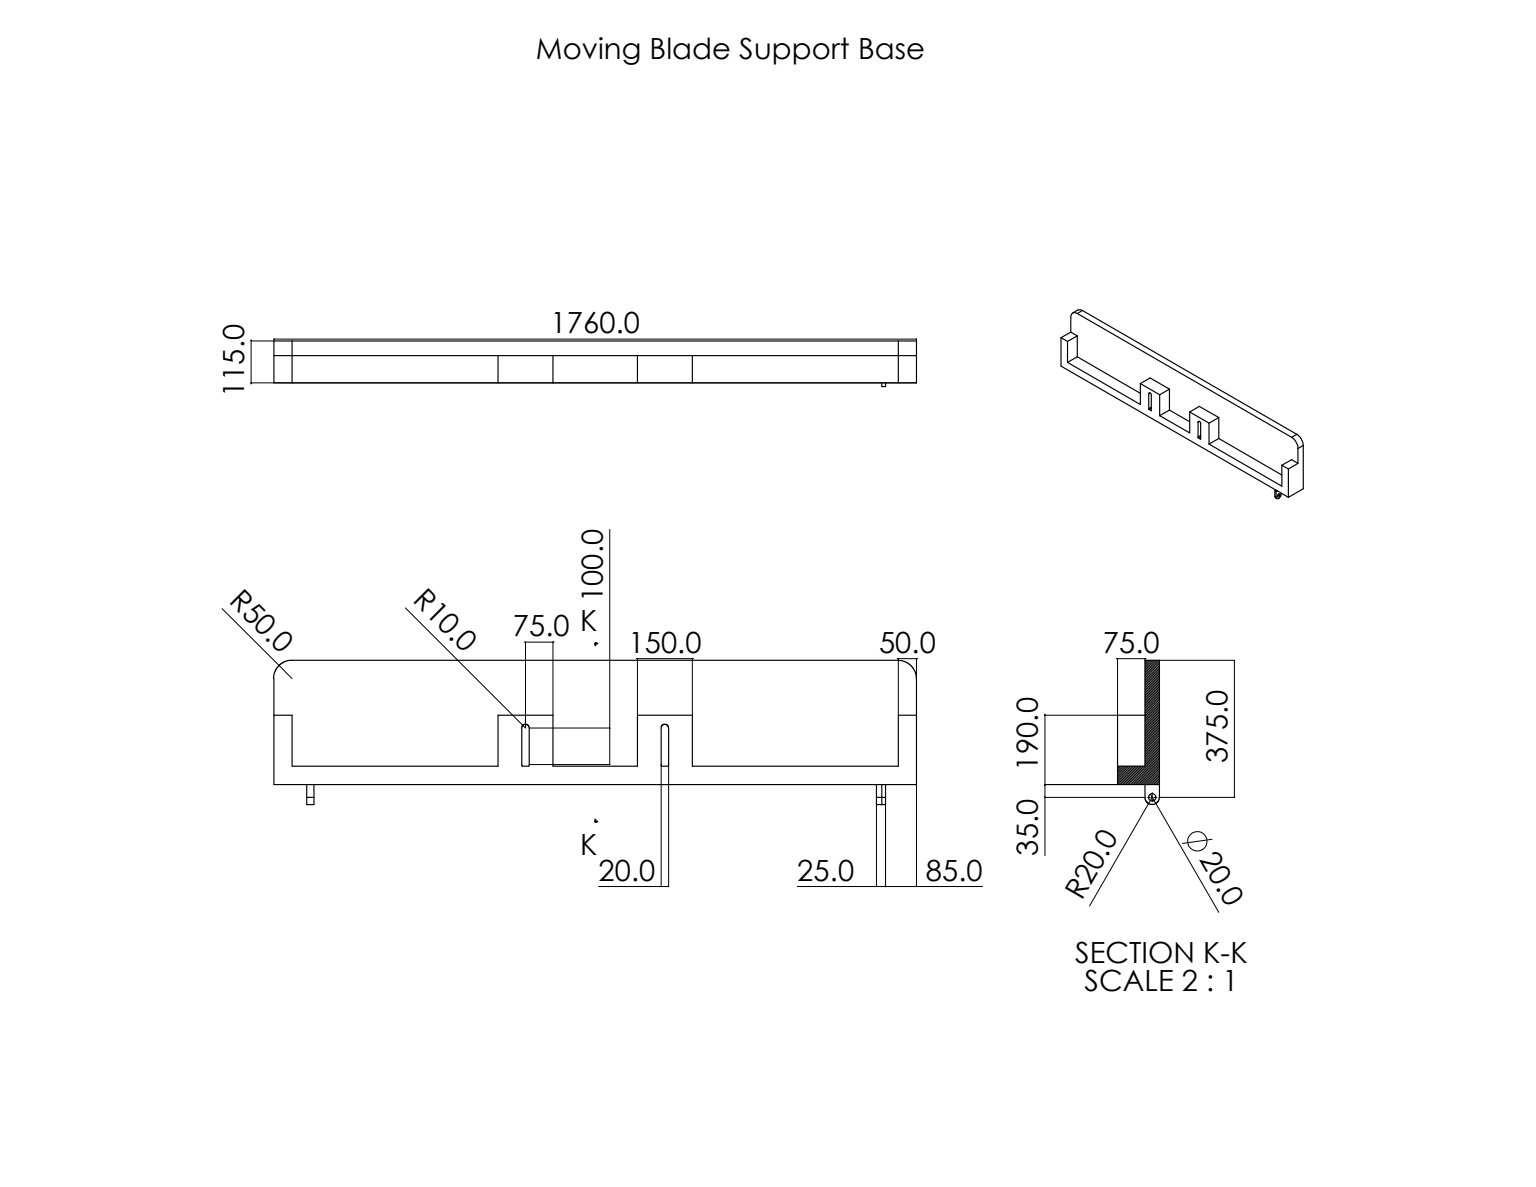
ISO-10303-21;
HEADER;
FILE_DESCRIPTION (('STEP AP214'),
    '1' );
FILE_NAME ('Moving Blade Support Base.step',
    '2026-10-21T17:07:05',
    ( '' ),
    ( '' ),
    'SwSTEP 2.0',
    'SolidWorks 2025',
    '' );
FILE_SCHEMA (( 'AUTOMOTIVE_DESIGN' ));
ENDSEC;

DATA;
#66=VERTEX_POINT ( 'NONE', #43052 ) ;
#76=DIRECTION ( 'NONE',  ( 1.000000000000000000, -5.551115123125783688E-16, 0.000000000000000000 ) ) ;
#92=DIRECTION ( 'NONE',  ( -1.000000000000000000, 0.000000000000000000, 0.000000000000000000 ) ) ;
#114=EDGE_CURVE ( 'NONE', #22938, #120, #8459, .T. ) ;
#120=VERTEX_POINT ( 'NONE', #34001 ) ;
#189=ADVANCED_FACE ( 'NONE', ( #37479 ), #13000, .F. ) ;
#193=CARTESIAN_POINT ( 'NONE',  ( -879.9999999999992042, 529.9999999999997726, -360.0000000000000000 ) ) ;
#205=EDGE_LOOP ( 'NONE', ( #30686, #19358, #44949, #34895 ) ) ;
#289=EDGE_LOOP ( 'NONE', ( #32622, #40266, #14008, #33528 ) ) ;
#307=DIRECTION ( 'NONE',  ( 1.000000000000000000, 0.000000000000000000, -0.000000000000000000 ) ) ;
#369=CARTESIAN_POINT ( 'NONE',  ( 200.7583438952259485, 394.6698570112193920, -274.9999999999999432 ) ) ;
#380=VECTOR ( 'NONE', #7221, 1000.000000000000000 ) ;
#396=AXIS2_PLACEMENT_3D ( 'NONE', #5672, #19302, #1519 ) ;
#398=CARTESIAN_POINT ( 'NONE',  ( -769.9999999999992042, 205.0000000000000568, -329.9999999999999432 ) ) ;
#404=FACE_OUTER_BOUND ( 'NONE', #21934, .T. ) ;
#412=VECTOR ( 'NONE', #33820, 1000.000000000000000 ) ;
#435=AXIS2_PLACEMENT_3D ( 'NONE', #25066, #43082, #39180 ) ;
#520=VECTOR ( 'NONE', #16329, 1000.000000000000000 ) ;
#539=ORIENTED_EDGE ( 'NONE', *, *, #26142, .F. ) ;
#553=LINE ( 'NONE', #7485, #44537 ) ;
#616=LINE ( 'NONE', #11017, #6169 ) ;
#637=VERTEX_POINT ( 'NONE', #20374 ) ;
#689=EDGE_CURVE ( 'NONE', #12562, #45491, #45323, .T. ) ;
#735=LINE ( 'NONE', #4212, #45701 ) ;
#784=CARTESIAN_POINT ( 'NONE',  ( 1238.921997096861332, 430.0000000000002842, -320.0000000000000568 ) ) ;
#829=LINE ( 'NONE', #22074, #26924 ) ;
#847=LINE ( 'NONE', #398, #9226 ) ;
#856=ORIENTED_EDGE ( 'NONE', *, *, #1291, .T. ) ;
#876=DIRECTION ( 'NONE',  ( -0.000000000000000000, -0.000000000000000000, 1.000000000000000000 ) ) ;
#879=DIRECTION ( 'NONE',  ( -0.000000000000000000, 1.000000000000000000, -0.000000000000000000 ) ) ;
#904=ORIENTED_EDGE ( 'NONE', *, *, #41975, .F. ) ;
#921=ORIENTED_EDGE ( 'NONE', *, *, #22135, .T. ) ;
#945=DIRECTION ( 'NONE',  ( 1.000000000000000000, 0.000000000000000000, 0.000000000000000000 ) ) ;
#983=FACE_OUTER_BOUND ( 'NONE', #35453, .T. ) ;
#1014=EDGE_CURVE ( 'NONE', #33458, #19810, #12588, .T. ) ;
#1053=CARTESIAN_POINT ( 'NONE',  ( -829.9999999999992042, 529.9999999999997726, -244.9999999999999716 ) ) ;
#1065=DIRECTION ( 'NONE',  ( 0.000000000000000000, 0.000000000000000000, 1.000000000000000000 ) ) ;
#1108=FACE_OUTER_BOUND ( 'NONE', #17628, .T. ) ;
#1137=AXIS2_PLACEMENT_3D ( 'NONE', #35687, #24841, #32239 ) ;
#1145=ORIENTED_EDGE ( 'NONE', *, *, #10271, .T. ) ;
#1157=ORIENTED_EDGE ( 'NONE', *, *, #3258, .T. ) ;
#1172=DIRECTION ( 'NONE',  ( 0.000000000000000000, 0.000000000000000000, -1.000000000000000000 ) ) ;
#1228=DIRECTION ( 'NONE',  ( 0.000000000000000000, 0.000000000000000000, -1.000000000000000000 ) ) ;
#1241=EDGE_LOOP ( 'NONE', ( #15487, #34240, #2964, #23570 ) ) ;
#1291=EDGE_CURVE ( 'NONE', #23098, #22606, #40548, .T. ) ;
#1294=DIRECTION ( 'NONE',  ( -0.000000000000000000, -4.857225732735055920E-15, 1.000000000000000000 ) ) ;
#1337=CARTESIAN_POINT ( 'NONE',  ( -769.9999999999992042, 205.0000000000000568, -339.9999999999999432 ) ) ;
#1348=VECTOR ( 'NONE', #24622, 1000.000000000000000 ) ;
#1386=FACE_OUTER_BOUND ( 'NONE', #24531, .T. ) ;
#1403=CARTESIAN_POINT ( 'NONE',  ( 1238.921997096861332, 240.0000000000000568, -244.9999999999999716 ) ) ;
#1470=CARTESIAN_POINT ( 'NONE',  ( -769.9999999999992042, 240.0000000000000568, -319.9999999999999432 ) ) ;
#1519=DIRECTION ( 'NONE',  ( 0.000000000000000000, 1.000000000000000000, 3.700743415417198493E-16 ) ) ;
#1552=CARTESIAN_POINT ( 'NONE',  ( 355.8971257818259915, 290.0000000000001137, -320.0000000000000568 ) ) ;
#1553=PLANE ( 'NONE',  #16394 ) ;
#1558=ADVANCED_FACE ( 'NONE', ( #21564 ), #18355, .F. ) ;
#1596=ORIENTED_EDGE ( 'NONE', *, *, #2120, .T. ) ;
#1603=PLANE ( 'NONE',  #28511 ) ;
#1607=ORIENTED_EDGE ( 'NONE', *, *, #1291, .F. ) ;
#1636=CARTESIAN_POINT ( 'NONE',  ( 1238.921997096861332, 430.0000000000002842, -244.9999999999999716 ) ) ;
#1637=VERTEX_POINT ( 'NONE', #36337 ) ;
#1647=VECTOR ( 'NONE', #23247, 1000.000000000000000 ) ;
#1656=VERTEX_POINT ( 'NONE', #25720 ) ;
#1673=AXIS2_PLACEMENT_3D ( 'NONE', #6623, #14021, #14713 ) ;
#1683=ADVANCED_FACE ( 'NONE', ( #32198 ), #25251, .F. ) ;
#1700=ORIENTED_EDGE ( 'NONE', *, *, #30911, .T. ) ;
#1702=DIRECTION ( 'NONE',  ( 1.000000000000000000, 0.000000000000000000, 0.000000000000000000 ) ) ;
#1725=CARTESIAN_POINT ( 'NONE',  ( 789.9999999999992042, 205.0000000000000568, -339.9999999999999432 ) ) ;
#1735=EDGE_CURVE ( 'NONE', #2122, #26522, #22240, .T. ) ;
#1748=ORIENTED_EDGE ( 'NONE', *, *, #16779, .F. ) ;
#1785=DIRECTION ( 'NONE',  ( 1.000000000000000000, 0.000000000000000000, -0.000000000000000000 ) ) ;
#1804=EDGE_LOOP ( 'NONE', ( #9462, #35099, #17743, #26253, #8483, #37145 ) ) ;
#1822=AXIS2_PLACEMENT_3D ( 'NONE', #15835, #9132, #36861 ) ;
#1864=ORIENTED_EDGE ( 'NONE', *, *, #14216, .T. ) ;
#1876=ORIENTED_EDGE ( 'NONE', *, *, #25151, .T. ) ;
#1966=VECTOR ( 'NONE', #876, 1000.000000000000000 ) ;
#1986=AXIS2_PLACEMENT_3D ( 'NONE', #13107, #16800, #33423 ) ;
#1992=ORIENTED_EDGE ( 'NONE', *, *, #34285, .F. ) ;
#2027=DIRECTION ( 'NONE',  ( 0.000000000000000000, 0.000000000000000000, 1.000000000000000000 ) ) ;
#2035=ORIENTED_EDGE ( 'NONE', *, *, #26712, .F. ) ;
#2077=DIRECTION ( 'NONE',  ( 0.000000000000000000, 0.000000000000000000, -1.000000000000000000 ) ) ;
#2120=EDGE_CURVE ( 'NONE', #38502, #44613, #35364, .T. ) ;
#2122=VERTEX_POINT ( 'NONE', #30995 ) ;
#2134=ADVANCED_FACE ( 'NONE', ( #45556 ), #45093, .F. ) ;
#2152=CARTESIAN_POINT ( 'NONE',  ( 180.7583438952258348, 394.6698570112193920, -274.9999999999999432 ) ) ;
#2169=PLANE ( 'NONE',  #26255 ) ;
#2178=CARTESIAN_POINT ( 'NONE',  ( 265.7583438952258916, 430.0000000000002842, -244.9999999999999716 ) ) ;
#2191=LINE ( 'NONE', #16283, #28287 ) ;
#2255=VERTEX_POINT ( 'NONE', #13451 ) ;
#2316=( GEOMETRIC_REPRESENTATION_CONTEXT ( 3 ) GLOBAL_UNCERTAINTY_ASSIGNED_CONTEXT ( ( #45060 ) ) GLOBAL_UNIT_ASSIGNED_CONTEXT ( ( #37692, #10198, #13223 ) ) REPRESENTATION_CONTEXT ( 'NONE', 'WORKASPACE' ) );
#2317=DIRECTION ( 'NONE',  ( 0.000000000000000000, -0.000000000000000000, 1.000000000000000000 ) ) ;
#2321=ORIENTED_EDGE ( 'NONE', *, *, #12855, .F. ) ;
#2355=DIRECTION ( 'NONE',  ( 0.000000000000000000, 0.000000000000000000, 1.000000000000000000 ) ) ;
#2374=ORIENTED_EDGE ( 'NONE', *, *, #14579, .T. ) ;
#2390=CARTESIAN_POINT ( 'NONE',  ( -200.7583438952258916, 294.6698570112193920, -274.9999999999999432 ) ) ;
#2394=CARTESIAN_POINT ( 'NONE',  ( -769.9999999999992042, 205.0000000000000568, -350.0000000000000000 ) ) ;
#2396=EDGE_LOOP ( 'NONE', ( #22146, #5273, #24875, #15758, #2484, #37091 ) ) ;
#2399=DIRECTION ( 'NONE',  ( -1.000000000000000000, 0.000000000000000000, 0.000000000000000000 ) ) ;
#2403=FACE_OUTER_BOUND ( 'NONE', #14861, .T. ) ;
#2473=LINE ( 'NONE', #38499, #1348 ) ;
#2484=ORIENTED_EDGE ( 'NONE', *, *, #4345, .T. ) ;
#2490=AXIS2_PLACEMENT_3D ( 'NONE', #11634, #39134, #42812 ) ;
#2569=CARTESIAN_POINT ( 'NONE',  ( 794.9999999999993179, 240.0000000000000853, -275.0000000000000000 ) ) ;
#2580=CARTESIAN_POINT ( 'NONE',  ( 784.9999999999992042, 205.0000000000000568, -255.0000000000000000 ) ) ;
#2594=VECTOR ( 'NONE', #24062, 1000.000000000000000 ) ;
#2601=FACE_OUTER_BOUND ( 'NONE', #38457, .T. ) ;
#2619=VERTEX_POINT ( 'NONE', #14363 ) ;
#2644=LINE ( 'NONE', #5407, #3910 ) ;
#2662=ADVANCED_FACE ( 'NONE', ( #28443 ), #42759, .T. ) ;
#2666=ADVANCED_FACE ( 'NONE', ( #14610 ), #43216, .F. ) ;
#2669=ORIENTED_EDGE ( 'NONE', *, *, #27519, .F. ) ;
#2752=EDGE_LOOP ( 'NONE', ( #5471, #20327, #25171, #15457 ) ) ;
#2797=ORIENTED_EDGE ( 'NONE', *, *, #18532, .T. ) ;
#2850=( NAMED_UNIT ( * ) PLANE_ANGLE_UNIT ( ) SI_UNIT ( $, .RADIAN. ) );
#2853=ORIENTED_EDGE ( 'NONE', *, *, #4945, .F. ) ;
#2878=FACE_OUTER_BOUND ( 'NONE', #35462, .T. ) ;
#2898=ADVANCED_FACE ( 'NONE', ( #5539, #37640, #18973 ), #40216, .F. ) ;
#2909=EDGE_CURVE ( 'NONE', #33022, #33694, #40657, .T. ) ;
#2964=ORIENTED_EDGE ( 'NONE', *, *, #13105, .F. ) ;
#3014=ORIENTED_EDGE ( 'NONE', *, *, #18532, .F. ) ;
#3081=DIRECTION ( 'NONE',  ( 0.000000000000000000, 0.000000000000000000, -1.000000000000000000 ) ) ;
#3082=DIRECTION ( 'NONE',  ( -0.000000000000000000, -0.000000000000000000, 1.000000000000000000 ) ) ;
#3087=VERTEX_POINT ( 'NONE', #20084 ) ;
#3094=LINE ( 'NONE', #34515, #5316 ) ;
#3171=VERTEX_POINT ( 'NONE', #6468 ) ;
#3254=CIRCLE ( 'NONE', #2490, 10.00000000000000888 ) ;
#3258=EDGE_CURVE ( 'NONE', #37112, #36817, #13621, .T. ) ;
#3270=AXIS2_PLACEMENT_3D ( 'NONE', #10948, #20633, #307 ) ;
#3325=EDGE_LOOP ( 'NONE', ( #12467, #24130 ) ) ;
#3330=DIRECTION ( 'NONE',  ( -1.000000000000000000, 0.000000000000000000, 0.000000000000000000 ) ) ;
#3343=CARTESIAN_POINT ( 'NONE',  ( 180.7583438952260622, 239.9999999999991473, -244.9999999999999716 ) ) ;
#3384=ORIENTED_EDGE ( 'NONE', *, *, #14831, .F. ) ;
#3479=EDGE_CURVE ( 'NONE', #34504, #21916, #14994, .T. ) ;
#3487=AXIS2_PLACEMENT_3D ( 'NONE', #27406, #9632, #8946 ) ;
#3553=ORIENTED_EDGE ( 'NONE', *, *, #6505, .F. ) ;
#3570=DIRECTION ( 'NONE',  ( 0.000000000000000000, 0.000000000000000000, -1.000000000000000000 ) ) ;
#3595=ORIENTED_EDGE ( 'NONE', *, *, #14216, .F. ) ;
#3605=AXIS2_PLACEMENT_3D ( 'NONE', #14612, #17604, #28446 ) ;
#3661=VECTOR ( 'NONE', #15436, 1000.000000000000000 ) ;
#3682=EDGE_LOOP ( 'NONE', ( #18165, #4144, #29968, #9995, #14865, #36556 ) ) ;
#3691=CARTESIAN_POINT ( 'NONE',  ( 355.8971257818259915, 290.0000000000001137, -244.9999999999999716 ) ) ;
#3754=ORIENTED_EDGE ( 'NONE', *, *, #38002, .F. ) ;
#3763=ORIENTED_EDGE ( 'NONE', *, *, #42223, .T. ) ;
#3805=DIRECTION ( 'NONE',  ( -0.000000000000000000, -0.000000000000000000, 1.000000000000000000 ) ) ;
#3892=ORIENTED_EDGE ( 'NONE', *, *, #42510, .F. ) ;
#3894=CARTESIAN_POINT ( 'NONE',  ( -829.9999999999994316, 579.9999999999998863, -360.0000000000000000 ) ) ;
#3910=VECTOR ( 'NONE', #13045, 1000.000000000000000 ) ;
#3938=VECTOR ( 'NONE', #20737, 1000.000000000000000 ) ;
#4027=EDGE_CURVE ( 'NONE', #37165, #1637, #32526, .T. ) ;
#4085=CARTESIAN_POINT ( 'NONE',  ( -789.9999999999992042, 205.0000000000000568, -350.0000000000000000 ) ) ;
#4086=FACE_OUTER_BOUND ( 'NONE', #29358, .T. ) ;
#4112=EDGE_CURVE ( 'NONE', #32155, #33694, #39924, .T. ) ;
#4114=EDGE_CURVE ( 'NONE', #1656, #27668, #11278, .T. ) ;
#4144=ORIENTED_EDGE ( 'NONE', *, *, #30071, .T. ) ;
#4202=CARTESIAN_POINT ( 'NONE',  ( -200.7583438952259485, 394.6698570112193920, -274.9999999999999432 ) ) ;
#4212=CARTESIAN_POINT ( 'NONE',  ( 794.9999999999993179, 205.0000000000000568, -274.9999999999999432 ) ) ;
#4234=ORIENTED_EDGE ( 'NONE', *, *, #22360, .F. ) ;
#4253=DIRECTION ( 'NONE',  ( 0.000000000000000000, 0.000000000000000000, 1.000000000000000000 ) ) ;
#4345=EDGE_CURVE ( 'NONE', #66, #19810, #34259, .T. ) ;
#4385=EDGE_CURVE ( 'NONE', #42899, #637, #19732, .T. ) ;
#4463=VERTEX_POINT ( 'NONE', #37740 ) ;
#4471=ORIENTED_EDGE ( 'NONE', *, *, #27831, .T. ) ;
#4532=LINE ( 'NONE', #22295, #34179 ) ;
#4546=ORIENTED_EDGE ( 'NONE', *, *, #26712, .T. ) ;
#4581=EDGE_CURVE ( 'NONE', #22016, #14103, #43589, .T. ) ;
#4627=EDGE_LOOP ( 'NONE', ( #36019, #24779, #36652, #33925, #45163, #24094 ) ) ;
#4685=DIRECTION ( 'NONE',  ( 1.000000000000000000, 0.000000000000000000, 0.000000000000000000 ) ) ;
#4731=ORIENTED_EDGE ( 'NONE', *, *, #1735, .F. ) ;
#4737=LINE ( 'NONE', #25067, #39541 ) ;
#4746=LINE ( 'NONE', #39656, #17406 ) ;
#4767=CARTESIAN_POINT ( 'NONE',  ( 1238.921997096861332, 240.0000000000000568, -244.9999999999999716 ) ) ;
#4776=EDGE_LOOP ( 'NONE', ( #38412, #25645 ) ) ;
#4803=LINE ( 'NONE', #26272, #24105 ) ;
#4804=DIRECTION ( 'NONE',  ( 1.000000000000000000, 0.000000000000000000, -0.000000000000000000 ) ) ;
#4815=AXIS2_PLACEMENT_3D ( 'NONE', #27835, #17202, #41930 ) ;
#4849=ORIENTED_EDGE ( 'NONE', *, *, #38917, .F. ) ;
#4857=ORIENTED_EDGE ( 'NONE', *, *, #3479, .F. ) ;
#4871=DIRECTION ( 'NONE',  ( -0.000000000000000000, -0.000000000000000000, 1.000000000000000000 ) ) ;
#4877=ADVANCED_FACE ( 'NONE', ( #21106 ), #42118, .T. ) ;
#4945=EDGE_CURVE ( 'NONE', #40516, #41324, #35818, .T. ) ;
#4955=ORIENTED_EDGE ( 'NONE', *, *, #28981, .F. ) ;
#4986=CARTESIAN_POINT ( 'NONE',  ( -265.7583438952258916, 430.0000000000002842, -244.9999999999999716 ) ) ;
#5011=EDGE_LOOP ( 'NONE', ( #3763, #40780, #25792, #15417 ) ) ;
#5037=CARTESIAN_POINT ( 'NONE',  ( -200.7583438952259485, 394.6698570112193920, -274.9999999999999432 ) ) ;
#5113=EDGE_CURVE ( 'NONE', #11672, #33458, #33310, .T. ) ;
#5137=ORIENTED_EDGE ( 'NONE', *, *, #25151, .F. ) ;
#5143=DIRECTION ( 'NONE',  ( -1.000000000000000000, -0.000000000000000000, -0.000000000000000000 ) ) ;
#5214=FACE_OUTER_BOUND ( 'NONE', #22702, .T. ) ;
#5223=ORIENTED_EDGE ( 'NONE', *, *, #1014, .T. ) ;
#5273=ORIENTED_EDGE ( 'NONE', *, *, #37945, .T. ) ;
#5274=ORIENTED_EDGE ( 'NONE', *, *, #22162, .T. ) ;
#5312=LINE ( 'NONE', #5543, #10273 ) ;
#5316=VECTOR ( 'NONE', #28249, 1000.000000000000000 ) ;
#5357=CARTESIAN_POINT ( 'NONE',  ( 794.9999999999993179, 239.9999999999998863, -235.0000000000000000 ) ) ;
#5380=CYLINDRICAL_SURFACE ( 'NONE', #27823, 20.00000000000001776 ) ;
#5381=ORIENTED_EDGE ( 'NONE', *, *, #14831, .T. ) ;
#5389=VERTEX_POINT ( 'NONE', #44381 ) ;
#5395=VERTEX_POINT ( 'NONE', #37913 ) ;
#5407=CARTESIAN_POINT ( 'NONE',  ( 769.9999999999992042, 240.0000000000000568, -319.9999999999999432 ) ) ;
#5428=PLANE ( 'NONE',  #396 ) ;
#5463=CARTESIAN_POINT ( 'NONE',  ( -829.9999999999992042, 290.0000000000001137, -244.9999999999999716 ) ) ;
#5471=ORIENTED_EDGE ( 'NONE', *, *, #42213, .F. ) ;
#5534=AXIS2_PLACEMENT_3D ( 'NONE', #41405, #23598, #27312 ) ;
#5539=FACE_BOUND ( 'NONE', #4627, .T. ) ;
#5543=CARTESIAN_POINT ( 'NONE',  ( 265.7583438952258916, 430.0000000000002842, -320.0000000000000000 ) ) ;
#5563=FACE_OUTER_BOUND ( 'NONE', #6612, .T. ) ;
#5593=CIRCLE ( 'NONE', #34347, 50.00000000000004263 ) ;
#5618=LINE ( 'NONE', #2152, #15309 ) ;
#5623=VECTOR ( 'NONE', #27450, 1000.000000000000000 ) ;
#5634=DIRECTION ( 'NONE',  ( -0.000000000000000000, 1.586032892321651891E-15, 1.000000000000000000 ) ) ;
#5644=CYLINDRICAL_SURFACE ( 'NONE', #32254, 50.00000000000004263 ) ;
#5660=VECTOR ( 'NONE', #41163, 1000.000000000000000 ) ;
#5672=CARTESIAN_POINT ( 'NONE',  ( 1238.921997096861332, 579.9999999999998863, -320.0000000000000000 ) ) ;
#5711=LINE ( 'NONE', #16106, #19361 ) ;
#5723=ORIENTED_EDGE ( 'NONE', *, *, #38818, .F. ) ;
#5754=EDGE_LOOP ( 'NONE', ( #16476, #10279, #856, #4471 ) ) ;
#5826=AXIS2_PLACEMENT_3D ( 'NONE', #9700, #16399, #44345 ) ;
#5873=DIRECTION ( 'NONE',  ( -1.000000000000000000, -0.000000000000000000, -0.000000000000000000 ) ) ;
#5902=ORIENTED_EDGE ( 'NONE', *, *, #24394, .F. ) ;
#5908=ORIENTED_EDGE ( 'NONE', *, *, #40798, .F. ) ;
#5926=PLANE ( 'NONE',  #21172 ) ;
#5947=DIRECTION ( 'NONE',  ( 0.000000000000000000, -0.000000000000000000, -1.000000000000000000 ) ) ;
#5991=DIRECTION ( 'NONE',  ( -0.000000000000000000, 1.000000000000000000, -1.586032892321652088E-15 ) ) ;
#6069=VECTOR ( 'NONE', #20486, 1000.000000000000000 ) ;
#6071=DIRECTION ( 'NONE',  ( 0.000000000000000000, 0.000000000000000000, -1.000000000000000000 ) ) ;
#6075=DIRECTION ( 'NONE',  ( 1.000000000000000000, 0.000000000000000000, 0.000000000000000000 ) ) ;
#6080=VECTOR ( 'NONE', #21557, 1000.000000000000000 ) ;
#6100=DIRECTION ( 'NONE',  ( 0.000000000000000000, -0.000000000000000000, -1.000000000000000000 ) ) ;
#6109=LINE ( 'NONE', #3343, #30527 ) ;
#6152=VECTOR ( 'NONE', #6590, 1000.000000000000000 ) ;
#6166=CARTESIAN_POINT ( 'NONE',  ( -879.9999999999992042, 529.9999999999997726, -320.0000000000000000 ) ) ;
#6169=VECTOR ( 'NONE', #25084, 1000.000000000000000 ) ;
#6188=LINE ( 'NONE', #17048, #15072 ) ;
#6217=CIRCLE ( 'NONE', #40164, 20.00000000000001776 ) ;
#6246=CARTESIAN_POINT ( 'NONE',  ( 355.8971257818259915, 290.0000000000001137, -244.9999999999999716 ) ) ;
#6263=CARTESIAN_POINT ( 'NONE',  ( 829.9999999999992042, -600.0000000000000000, -320.0000000000000568 ) ) ;
#6282=VECTOR ( 'NONE', #33387, 1000.000000000000000 ) ;
#6286=EDGE_CURVE ( 'NONE', #36310, #21150, #26154, .T. ) ;
#6312=( NAMED_UNIT ( * ) SI_UNIT ( $, .STERADIAN. ) SOLID_ANGLE_UNIT ( ) );
#6333=FACE_BOUND ( 'NONE', #3325, .T. ) ;
#6374=ADVANCED_FACE ( 'NONE', ( #2878, #6567 ), #21116, .F. ) ;
#6383=VERTEX_POINT ( 'NONE', #41914 ) ;
#6452=DIRECTION ( 'NONE',  ( 0.000000000000000000, 0.000000000000000000, -1.000000000000000000 ) ) ;
#6467=LINE ( 'NONE', #17307, #41700 ) ;
#6468=CARTESIAN_POINT ( 'NONE',  ( -879.9999999999992042, 430.0000000000002842, -320.0000000000000568 ) ) ;
#6491=AXIS2_PLACEMENT_3D ( 'NONE', #40901, #32850, #9271 ) ;
#6505=EDGE_CURVE ( 'NONE', #8476, #15857, #24555, .T. ) ;
#6527=DIRECTION ( 'NONE',  ( 0.000000000000000000, 0.000000000000000000, 1.000000000000000000 ) ) ;
#6536=VERTEX_POINT ( 'NONE', #41685 ) ;
#6546=VECTOR ( 'NONE', #14134, 1000.000000000000000 ) ;
#6567=FACE_BOUND ( 'NONE', #38886, .T. ) ;
#6590=DIRECTION ( 'NONE',  ( -0.000000000000000000, -1.000000000000000000, -0.000000000000000000 ) ) ;
#6607=EDGE_CURVE ( 'NONE', #19810, #3171, #35887, .T. ) ;
#6612=EDGE_LOOP ( 'NONE', ( #15855, #29638, #34728, #12062 ) ) ;
#6616=VECTOR ( 'NONE', #38203, 1000.000000000000000 ) ;
#6623=CARTESIAN_POINT ( 'NONE',  ( 190.7583438952258916, 294.6698570112193920, -244.9999999999999716 ) ) ;
#6674=EDGE_LOOP ( 'NONE', ( #23150, #24484, #26874, #15076 ) ) ;
#6684=CARTESIAN_POINT ( 'NONE',  ( 784.9999999999992042, 240.0000000000000853, -275.0000000000000000 ) ) ;
#6689=CARTESIAN_POINT ( 'NONE',  ( -115.7583438952258774, 430.0000000000002842, -244.9999999999999716 ) ) ;
#6744=VECTOR ( 'NONE', #39080, 1000.000000000000000 ) ;
#6804=CARTESIAN_POINT ( 'NONE',  ( -789.9999999999992042, 205.0000000000000568, -319.9999999999999432 ) ) ;
#6842=LINE ( 'NONE', #7089, #44058 ) ;
#6894=DIRECTION ( 'NONE',  ( 0.000000000000000000, 0.000000000000000000, -1.000000000000000000 ) ) ;
#6928=VERTEX_POINT ( 'NONE', #5357 ) ;
#6933=AXIS2_PLACEMENT_3D ( 'NONE', #27413, #42413, #23702 ) ;
#6999=ORIENTED_EDGE ( 'NONE', *, *, #4385, .F. ) ;
#7012=CARTESIAN_POINT ( 'NONE',  ( 180.7583438952258916, 294.6698570112193920, -274.9999999999999432 ) ) ;
#7013=ORIENTED_EDGE ( 'NONE', *, *, #38114, .F. ) ;
#7043=VECTOR ( 'NONE', #26872, 1000.000000000000000 ) ;
#7056=LINE ( 'NONE', #42153, #20163 ) ;
#7089=CARTESIAN_POINT ( 'NONE',  ( -265.7583438952258916, 290.0000000000001705, -320.0000000000000000 ) ) ;
#7096=DIRECTION ( 'NONE',  ( -1.000000000000000000, 0.000000000000000000, 0.000000000000000000 ) ) ;
#7173=EDGE_LOOP ( 'NONE', ( #5274, #37675, #45424, #10452 ) ) ;
#7221=DIRECTION ( 'NONE',  ( -0.000000000000000000, -0.000000000000000000, 1.000000000000000000 ) ) ;
#7247=EDGE_CURVE ( 'NONE', #44144, #37112, #40704, .T. ) ;
#7261=ORIENTED_EDGE ( 'NONE', *, *, #45035, .F. ) ;
#7302=ORIENTED_EDGE ( 'NONE', *, *, #38540, .T. ) ;
#7309=DIRECTION ( 'NONE',  ( 0.000000000000000000, 0.000000000000000000, -1.000000000000000000 ) ) ;
#7310=FACE_OUTER_BOUND ( 'NONE', #16254, .T. ) ;
#7328=CARTESIAN_POINT ( 'NONE',  ( -769.9999999999992042, 205.0000000000000568, -339.9999999999999432 ) ) ;
#7333=FACE_OUTER_BOUND ( 'NONE', #5754, .T. ) ;
#7367=CARTESIAN_POINT ( 'NONE',  ( 789.9999999999992042, 205.0000000000000568, -360.0000000000000000 ) ) ;
#7373=ORIENTED_EDGE ( 'NONE', *, *, #6505, .T. ) ;
#7421=ORIENTED_EDGE ( 'NONE', *, *, #24171, .F. ) ;
#7469=VERTEX_POINT ( 'NONE', #28202 ) ;
#7473=EDGE_CURVE ( 'NONE', #12764, #32851, #24501, .T. ) ;
#7476=CARTESIAN_POINT ( 'NONE',  ( 794.9999999999993179, 239.9999999999998863, -235.0000000000000000 ) ) ;
#7485=CARTESIAN_POINT ( 'NONE',  ( 829.9999999999992042, 430.0000000000002842, -320.0000000000000568 ) ) ;
#7530=DIRECTION ( 'NONE',  ( 0.000000000000000000, 0.000000000000000000, -1.000000000000000000 ) ) ;
#7531=DIRECTION ( 'NONE',  ( -0.000000000000000000, 1.000000000000000000, 6.938893903907241197E-16 ) ) ;
#7544=DIRECTION ( 'NONE',  ( -1.000000000000000000, -8.326672684688676025E-16, 0.000000000000000000 ) ) ;
#7575=VERTEX_POINT ( 'NONE', #37695 ) ;
#7611=CARTESIAN_POINT ( 'NONE',  ( 265.7583438952258916, 290.0000000000001137, -320.0000000000000568 ) ) ;
#7747=VERTEX_POINT ( 'NONE', #35584 ) ;
#7789=AXIS2_PLACEMENT_3D ( 'NONE', #7328, #7096, #34399 ) ;
#7833=DIRECTION ( 'NONE',  ( -0.000000000000000000, 1.000000000000000000, -0.000000000000000000 ) ) ;
#7838=CIRCLE ( 'NONE', #38823, 10.00000000000000888 ) ;
#7849=DIRECTION ( 'NONE',  ( -1.000000000000000000, -0.000000000000000000, -0.000000000000000000 ) ) ;
#7937=EDGE_LOOP ( 'NONE', ( #28588, #37208, #32066, #23296 ) ) ;
#7952=LINE ( 'NONE', #43032, #8407 ) ;
#7998=DIRECTION ( 'NONE',  ( 1.000000000000000000, -0.000000000000000000, -0.000000000000000000 ) ) ;
#8057=CARTESIAN_POINT ( 'NONE',  ( -265.7583438952258916, -600.0000000000000000, -320.0000000000000000 ) ) ;
#8082=LINE ( 'NONE', #11980, #37938 ) ;
#8131=EDGE_CURVE ( 'NONE', #16382, #12764, #34405, .T. ) ;
#8171=LINE ( 'NONE', #43485, #6080 ) ;
#8204=VERTEX_POINT ( 'NONE', #38113 ) ;
#8226=CARTESIAN_POINT ( 'NONE',  ( 879.9999999999992042, 240.0000000000000568, -244.9999999999999716 ) ) ;
#8274=EDGE_CURVE ( 'NONE', #31293, #5389, #6467, .T. ) ;
#8328=VECTOR ( 'NONE', #17490, 1000.000000000000000 ) ;
#8368=ORIENTED_EDGE ( 'NONE', *, *, #26992, .F. ) ;
#8378=LINE ( 'NONE', #12070, #36619 ) ;
#8407=VECTOR ( 'NONE', #11396, 1000.000000000000000 ) ;
#8421=VERTEX_POINT ( 'NONE', #9476 ) ;
#8428=ORIENTED_EDGE ( 'NONE', *, *, #34615, .F. ) ;
#8459=CIRCLE ( 'NONE', #34244, 10.00000000000006395 ) ;
#8476=VERTEX_POINT ( 'NONE', #33204 ) ;
#8483=ORIENTED_EDGE ( 'NONE', *, *, #44416, .T. ) ;
#8503=CARTESIAN_POINT ( 'NONE',  ( 265.7583438952258916, -600.0000000000000000, -244.9999999999999716 ) ) ;
#8540=ORIENTED_EDGE ( 'NONE', *, *, #1014, .F. ) ;
#8601=ORIENTED_EDGE ( 'NONE', *, *, #23000, .T. ) ;
#8619=CARTESIAN_POINT ( 'NONE',  ( -829.9999999999992042, -600.0000000000000000, -244.9999999999995168 ) ) ;
#8644=AXIS2_PLACEMENT_3D ( 'NONE', #7476, #35628, #32182 ) ;
#8657=ORIENTED_EDGE ( 'NONE', *, *, #42213, .T. ) ;
#8665=ORIENTED_EDGE ( 'NONE', *, *, #17723, .T. ) ;
#8703=CARTESIAN_POINT ( 'NONE',  ( 1238.921997096861332, 240.0000000000000853, -360.0000000000000000 ) ) ;
#8742=CYLINDRICAL_SURFACE ( 'NONE', #18710, 10.00000000000000888 ) ;
#8871=ORIENTED_EDGE ( 'NONE', *, *, #15402, .F. ) ;
#8900=FACE_OUTER_BOUND ( 'NONE', #2396, .T. ) ;
#8920=EDGE_LOOP ( 'NONE', ( #921, #1748, #23517, #35732 ) ) ;
#8922=ADVANCED_FACE ( 'NONE', ( #13784 ), #16789, .F. ) ;
#8926=EDGE_LOOP ( 'NONE', ( #5902, #20512, #35977, #20567, #33801, #30215 ) ) ;
#8941=LINE ( 'NONE', #23470, #18218 ) ;
#8946=DIRECTION ( 'NONE',  ( 0.000000000000000000, 0.000000000000000000, -1.000000000000000000 ) ) ;
#9031=VERTEX_POINT ( 'NONE', #38034 ) ;
#9039=CIRCLE ( 'NONE', #34852, 19.99999999999998934 ) ;
#9107=CARTESIAN_POINT ( 'NONE',  ( 180.7583438952258916, 294.6698570112193920, -274.9999999999999432 ) ) ;
#9132=DIRECTION ( 'NONE',  ( -0.000000000000000000, 1.000000000000000000, 0.000000000000000000 ) ) ;
#9136=EDGE_LOOP ( 'NONE', ( #44530, #32686, #26588, #20152, #28994, #40255, #11894, #45303, #1864, #16311, #5908, #22664, #25054, #38306 ) ) ;
#9154=ORIENTED_EDGE ( 'NONE', *, *, #34274, .T. ) ;
#9166=CARTESIAN_POINT ( 'NONE',  ( 784.9999999999992042, 239.9999999999998863, -235.0000000000000000 ) ) ;
#9172=AXIS2_PLACEMENT_3D ( 'NONE', #36324, #11391, #4685 ) ;
#9182=EDGE_CURVE ( 'NONE', #44613, #25018, #20235, .T. ) ;
#9226=VECTOR ( 'NONE', #14502, 1000.000000000000000 ) ;
#9253=LINE ( 'NONE', #12265, #37540 ) ;
#9271=DIRECTION ( 'NONE',  ( 0.000000000000000000, 0.000000000000000000, 1.000000000000000000 ) ) ;
#9287=LINE ( 'NONE', #6263, #43996 ) ;
#9320=ADVANCED_FACE ( 'NONE', ( #7310 ), #14225, .F. ) ;
#9326=VECTOR ( 'NONE', #39284, 1000.000000000000000 ) ;
#9337=CARTESIAN_POINT ( 'NONE',  ( 794.9999999999993179, 240.0000000000000853, -275.0000000000000000 ) ) ;
#9354=AXIS2_PLACEMENT_3D ( 'NONE', #24545, #31714, #38428 ) ;
#9422=VECTOR ( 'NONE', #15736, 1000.000000000000000 ) ;
#9431=EDGE_CURVE ( 'NONE', #4463, #22016, #4737, .T. ) ;
#9451=ORIENTED_EDGE ( 'NONE', *, *, #30318, .F. ) ;
#9462=ORIENTED_EDGE ( 'NONE', *, *, #27723, .T. ) ;
#9473=ADVANCED_FACE ( 'NONE', ( #39644 ), #38960, .F. ) ;
#9476=CARTESIAN_POINT ( 'NONE',  ( 784.9999999999992042, 205.0000000000000568, -245.0000000000000284 ) ) ;
#9498=ORIENTED_EDGE ( 'NONE', *, *, #33454, .F. ) ;
#9540=DIRECTION ( 'NONE',  ( 0.000000000000000000, 0.000000000000000000, 1.000000000000000000 ) ) ;
#9554=VECTOR ( 'NONE', #3082, 1000.000000000000000 ) ;
#9569=ORIENTED_EDGE ( 'NONE', *, *, #43347, .F. ) ;
#9581=DIRECTION ( 'NONE',  ( -0.000000000000000000, 1.000000000000000000, -0.000000000000000000 ) ) ;
#9632=DIRECTION ( 'NONE',  ( 1.000000000000000000, 0.000000000000000000, 0.000000000000000000 ) ) ;
#9638=CARTESIAN_POINT ( 'NONE',  ( -769.9999999999992042, 205.0000000000000568, -319.9999999999999432 ) ) ;
#9674=EDGE_LOOP ( 'NONE', ( #7421, #36199, #42960, #15361 ) ) ;
#9700=CARTESIAN_POINT ( 'NONE',  ( -190.7583438952258916, 294.6698570112193920, -244.9999999999999716 ) ) ;
#9724=ADVANCED_FACE ( 'NONE', ( #22945 ), #2169, .F. ) ;
#9770=CARTESIAN_POINT ( 'NONE',  ( 180.7583438952258348, 394.6698570112193920, -274.9999999999999432 ) ) ;
#9799=LINE ( 'NONE', #16053, #25297 ) ;
#9822=EDGE_LOOP ( 'NONE', ( #5137, #2321, #44202, #36220 ) ) ;
#9901=LINE ( 'NONE', #13840, #19641 ) ;
#9949=CIRCLE ( 'NONE', #15847, 19.99999999999998934 ) ;
#9953=CIRCLE ( 'NONE', #29152, 20.00000000000001776 ) ;
#9984=EDGE_CURVE ( 'NONE', #39117, #22606, #37331, .T. ) ;
#9995=ORIENTED_EDGE ( 'NONE', *, *, #35112, .F. ) ;
#10035=FACE_OUTER_BOUND ( 'NONE', #1241, .T. ) ;
#10049=AXIS2_PLACEMENT_3D ( 'NONE', #31512, #13279, #92 ) ;
#10082=DIRECTION ( 'NONE',  ( -0.000000000000000000, 0.000000000000000000, -1.000000000000000000 ) ) ;
#10094=VECTOR ( 'NONE', #43379, 1000.000000000000000 ) ;
#10175=DIRECTION ( 'NONE',  ( 1.000000000000000000, 0.000000000000000000, 0.000000000000000000 ) ) ;
#10179=VECTOR ( 'NONE', #18760, 1000.000000000000000 ) ;
#10198=( NAMED_UNIT ( * ) PLANE_ANGLE_UNIT ( ) SI_UNIT ( $, .RADIAN. ) );
#10204=VECTOR ( 'NONE', #44836, 1000.000000000000000 ) ;
#10217=CARTESIAN_POINT ( 'NONE',  ( -180.7583438952258348, 394.6698570112193920, -274.9999999999999432 ) ) ;
#10220=VERTEX_POINT ( 'NONE', #38653 ) ;
#10226=PLANE ( 'NONE',  #38925 ) ;
#10240=CARTESIAN_POINT ( 'NONE',  ( 794.9999999999993179, 205.0000000000000568, -255.0000000000000000 ) ) ;
#10271=EDGE_CURVE ( 'NONE', #2255, #36814, #32900, .T. ) ;
#10273=VECTOR ( 'NONE', #27260, 1000.000000000000000 ) ;
#10274=CARTESIAN_POINT ( 'NONE',  ( 769.9999999999992042, 205.0000000000000568, -339.9999999999999432 ) ) ;
#10276=ADVANCED_FACE ( 'NONE', ( #45361 ), #41895, .T. ) ;
#10279=ORIENTED_EDGE ( 'NONE', *, *, #15141, .F. ) ;
#10334=ORIENTED_EDGE ( 'NONE', *, *, #43836, .T. ) ;
#10445=ORIENTED_EDGE ( 'NONE', *, *, #41975, .T. ) ;
#10452=ORIENTED_EDGE ( 'NONE', *, *, #16779, .T. ) ;
#10477=DIRECTION ( 'NONE',  ( 0.000000000000000000, -1.000000000000000000, 0.000000000000000000 ) ) ;
#10535=CARTESIAN_POINT ( 'NONE',  ( 180.7583438952258348, 394.6698570112193920, -274.9999999999999432 ) ) ;
#10564=ADVANCED_FACE ( 'NONE', ( #25704 ), #22012, .F. ) ;
#10572=ORIENTED_EDGE ( 'NONE', *, *, #37945, .F. ) ;
#10629=AXIS2_PLACEMENT_3D ( 'NONE', #32436, #25492, #42820 ) ;
#10643=CARTESIAN_POINT ( 'NONE',  ( 265.7583438952258916, 290.0000000000001137, -244.9999999999999716 ) ) ;
#10657=VECTOR ( 'NONE', #43929, 1000.000000000000000 ) ;
#10662=DIRECTION ( 'NONE',  ( 0.000000000000000000, 0.000000000000000000, -1.000000000000000000 ) ) ;
#10715=CARTESIAN_POINT ( 'NONE',  ( 1238.921997096861332, 430.0000000000002842, -320.0000000000000568 ) ) ;
#10756=ORIENTED_EDGE ( 'NONE', *, *, #24413, .F. ) ;
#10829=CARTESIAN_POINT ( 'NONE',  ( 175.6195620086261613, 290.0000000000001137, -320.0000000000000568 ) ) ;
#10884=EDGE_CURVE ( 'NONE', #1637, #45115, #8378, .T. ) ;
#10898=CARTESIAN_POINT ( 'NONE',  ( 1238.921997096861332, 240.0000000000000568, -244.9999999999999716 ) ) ;
#10932=EDGE_LOOP ( 'NONE', ( #16729, #35225, #3892, #20497 ) ) ;
#10944=CARTESIAN_POINT ( 'NONE',  ( 200.7583438952259485, 394.6698570112193920, -274.9999999999999432 ) ) ;
#10948=CARTESIAN_POINT ( 'NONE',  ( 190.7583438952259485, 394.6698570112193920, -274.9999999999999432 ) ) ;
#10974=CARTESIAN_POINT ( 'NONE',  ( -115.7583438952258774, 430.0000000000002842, -244.9999999999999716 ) ) ;
#11017=CARTESIAN_POINT ( 'NONE',  ( 769.9999999999992042, 240.0000000000000568, -319.9999999999999432 ) ) ;
#11091=CARTESIAN_POINT ( 'NONE',  ( 794.9999999999993179, 205.0000000000000568, -265.0000000000000000 ) ) ;
#11092=ORIENTED_EDGE ( 'NONE', *, *, #22976, .T. ) ;
#11140=EDGE_CURVE ( 'NONE', #15121, #26522, #13214, .T. ) ;
#11150=EDGE_CURVE ( 'NONE', #14103, #7469, #9287, .T. ) ;
#11220=FACE_OUTER_BOUND ( 'NONE', #29159, .T. ) ;
#11225=LINE ( 'NONE', #369, #17442 ) ;
#11251=DIRECTION ( 'NONE',  ( -1.000000000000000000, -0.000000000000000000, -0.000000000000000000 ) ) ;
#11266=VERTEX_POINT ( 'NONE', #7367 ) ;
#11267=PRODUCT_CONTEXT ( 'NONE', #19019, 'mechanical' ) ;
#11278=LINE ( 'NONE', #42460, #11468 ) ;
#11336=ORIENTED_EDGE ( 'NONE', *, *, #44934, .F. ) ;
#11350=DIRECTION ( 'NONE',  ( 0.000000000000000000, 0.000000000000000000, 1.000000000000000000 ) ) ;
#11354=ADVANCED_FACE ( 'NONE', ( #22125 ), #36437, .F. ) ;
#11371=LINE ( 'NONE', #14388, #20500 ) ;
#11391=DIRECTION ( 'NONE',  ( 0.000000000000000000, -0.000000000000000000, -1.000000000000000000 ) ) ;
#11396=DIRECTION ( 'NONE',  ( -1.000000000000000000, -0.000000000000000000, -0.000000000000000000 ) ) ;
#11468=VECTOR ( 'NONE', #11513, 1000.000000000000000 ) ;
#11492=CARTESIAN_POINT ( 'NONE',  ( -115.7583438952258774, 430.0000000000002842, -320.0000000000000568 ) ) ;
#11513=DIRECTION ( 'NONE',  ( -1.000000000000000000, -0.000000000000000000, -0.000000000000000000 ) ) ;
#11532=ADVANCED_FACE ( 'NONE', ( #32999 ), #39927, .T. ) ;
#11590=DIRECTION ( 'NONE',  ( 0.000000000000000000, -0.000000000000000000, 1.000000000000000000 ) ) ;
#11611=EDGE_LOOP ( 'NONE', ( #1157, #43247, #14322, #40627, #27114 ) ) ;
#11618=EDGE_LOOP ( 'NONE', ( #25727, #21084, #38889, #43403 ) ) ;
#11634=CARTESIAN_POINT ( 'NONE',  ( 789.9999999999992042, 205.0000000000000568, -339.9999999999999432 ) ) ;
#11644=VECTOR ( 'NONE', #45117, 1000.000000000000000 ) ;
#11651=EDGE_CURVE ( 'NONE', #4463, #27157, #22571, .T. ) ;
#11672=VERTEX_POINT ( 'NONE', #14762 ) ;
#11726=EDGE_CURVE ( 'NONE', #43685, #21532, #44276, .T. ) ;
#11831=ORIENTED_EDGE ( 'NONE', *, *, #4114, .T. ) ;
#11894=ORIENTED_EDGE ( 'NONE', *, *, #18732, .F. ) ;
#11906=CYLINDRICAL_SURFACE ( 'NONE', #12706, 50.00000000000004263 ) ;
#11930=CIRCLE ( 'NONE', #28149, 10.00000000000000888 ) ;
#11931=EDGE_CURVE ( 'NONE', #11672, #8476, #30408, .T. ) ;
#11972=EDGE_CURVE ( 'NONE', #32155, #8476, #15873, .T. ) ;
#11980=CARTESIAN_POINT ( 'NONE',  ( -115.7583438952258774, 290.0000000000001705, -244.9999999999999716 ) ) ;
#12062=ORIENTED_EDGE ( 'NONE', *, *, #18732, .T. ) ;
#12070=CARTESIAN_POINT ( 'NONE',  ( -789.9999999999992042, 240.0000000000000568, -319.9999999999999432 ) ) ;
#12079=EDGE_CURVE ( 'NONE', #38375, #637, #35247, .T. ) ;
#12083=VECTOR ( 'NONE', #40338, 1000.000000000000000 ) ;
#12129=CARTESIAN_POINT ( 'NONE',  ( -829.9999999999992042, 430.0000000000002842, -319.9999999999996021 ) ) ;
#12132=DIRECTION ( 'NONE',  ( 0.000000000000000000, 0.000000000000000000, -1.000000000000000000 ) ) ;
#12164=EDGE_LOOP ( 'NONE', ( #43790, #21589, #34080, #36443 ) ) ;
#12168=AXIS2_PLACEMENT_3D ( 'NONE', #17679, #17447, #27370 ) ;
#12210=DIRECTION ( 'NONE',  ( 0.000000000000000000, -1.000000000000000000, 0.000000000000000000 ) ) ;
#12265=CARTESIAN_POINT ( 'NONE',  ( 879.9999999999992042, 579.9999999999998863, -320.0000000000000000 ) ) ;
#12268=VECTOR ( 'NONE', #25409, 1000.000000000000000 ) ;
#12283=FACE_BOUND ( 'NONE', #4776, .T. ) ;
#12294=ORIENTED_EDGE ( 'NONE', *, *, #44450, .T. ) ;
#12296=VECTOR ( 'NONE', #7833, 1000.000000000000000 ) ;
#12327=DIRECTION ( 'NONE',  ( -1.000000000000000000, 0.000000000000000000, 0.000000000000000000 ) ) ;
#12414=CARTESIAN_POINT ( 'NONE',  ( -879.9999999999992042, 579.9999999999998863, -360.0000000000000000 ) ) ;
#12422=CARTESIAN_POINT ( 'NONE',  ( 190.7583438952258916, 294.6698570112193920, -274.9999999999999432 ) ) ;
#12428=ORIENTED_EDGE ( 'NONE', *, *, #43078, .T. ) ;
#12447=VERTEX_POINT ( 'NONE', #25973 ) ;
#12463=CARTESIAN_POINT ( 'NONE',  ( 879.9999999999992042, 579.9999999999998863, -360.0000000000000000 ) ) ;
#12467=ORIENTED_EDGE ( 'NONE', *, *, #37644, .F. ) ;
#12474=CARTESIAN_POINT ( 'NONE',  ( 355.8971257818259915, 290.0000000000001137, -244.9999999999999716 ) ) ;
#12562=VERTEX_POINT ( 'NONE', #42862 ) ;
#12588=LINE ( 'NONE', #22966, #37250 ) ;
#12589=DIRECTION ( 'NONE',  ( 1.000000000000000000, -0.000000000000000000, 0.000000000000000000 ) ) ;
#12633=DIRECTION ( 'NONE',  ( 0.000000000000000000, -1.000000000000000000, 0.000000000000000000 ) ) ;
#12682=LINE ( 'NONE', #13605, #41557 ) ;
#12706=AXIS2_PLACEMENT_3D ( 'NONE', #1053, #25768, #21619 ) ;
#12736=PLANE ( 'NONE',  #37380 ) ;
#12764=VERTEX_POINT ( 'NONE', #28780 ) ;
#12802=CARTESIAN_POINT ( 'NONE',  ( 1238.921997096861332, 579.9999999999998863, -360.0000000000000000 ) ) ;
#12855=EDGE_CURVE ( 'NONE', #39585, #26480, #11225, .T. ) ;
#13000=PLANE ( 'NONE',  #5534 ) ;
#13009=ORIENTED_EDGE ( 'NONE', *, *, #39172, .F. ) ;
#13045=DIRECTION ( 'NONE',  ( 1.000000000000000000, 0.000000000000000000, 0.000000000000000000 ) ) ;
#13067=PLANE ( 'NONE',  #12168 ) ;
#13105=EDGE_CURVE ( 'NONE', #25018, #7575, #32934, .T. ) ;
#13107=CARTESIAN_POINT ( 'NONE',  ( -190.7583438952258916, 294.6698570112193920, -274.9999999999999432 ) ) ;
#13114=LINE ( 'NONE', #9638, #45250 ) ;
#13136=VERTEX_POINT ( 'NONE', #2394 ) ;
#13161=EDGE_LOOP ( 'NONE', ( #18940, #30114, #2853, #15354 ) ) ;
#13183=EDGE_CURVE ( 'NONE', #26065, #11266, #19963, .T. ) ;
#13199=PLANE ( 'NONE',  #35233 ) ;
#13214=LINE ( 'NONE', #39017, #43282 ) ;
#13223=( NAMED_UNIT ( * ) SI_UNIT ( $, .STERADIAN. ) SOLID_ANGLE_UNIT ( ) );
#13256=ORIENTED_EDGE ( 'NONE', *, *, #37668, .F. ) ;
#13263=DIRECTION ( 'NONE',  ( 0.000000000000000000, 0.000000000000000000, -1.000000000000000000 ) ) ;
#13279=DIRECTION ( 'NONE',  ( 0.000000000000000000, 0.000000000000000000, -1.000000000000000000 ) ) ;
#13329=LINE ( 'NONE', #44279, #520 ) ;
#13340=CARTESIAN_POINT ( 'NONE',  ( 190.7583438952258916, 294.6698570112193920, -244.9999999999999716 ) ) ;
#13342=DIRECTION ( 'NONE',  ( 0.000000000000000000, 0.000000000000000000, 1.000000000000000000 ) ) ;
#13350=CARTESIAN_POINT ( 'NONE',  ( 794.9999999999993179, 239.9999999999998863, -235.0000000000000000 ) ) ;
#13377=LINE ( 'NONE', #10829, #5623 ) ;
#13412=EDGE_CURVE ( 'NONE', #8421, #32576, #18929, .T. ) ;
#13414=ORIENTED_EDGE ( 'NONE', *, *, #35683, .F. ) ;
#13420=AXIS2_PLACEMENT_3D ( 'NONE', #2580, #24737, #1172 ) ;
#13451=CARTESIAN_POINT ( 'NONE',  ( 794.9999999999993179, 205.0000000000000568, -245.0000000000000284 ) ) ;
#13536=VECTOR ( 'NONE', #34578, 1000.000000000000000 ) ;
#13558=CARTESIAN_POINT ( 'NONE',  ( -199.6009925648704098, 290.0000000000001137, -274.9999999999999432 ) ) ;
#13586=DIRECTION ( 'NONE',  ( -1.000000000000000000, -0.000000000000000000, -0.000000000000000000 ) ) ;
#13604=PLANE ( 'NONE',  #32976 ) ;
#13605=CARTESIAN_POINT ( 'NONE',  ( 1238.921997096861332, 430.0000000000002842, -320.0000000000000568 ) ) ;
#13621=LINE ( 'NONE', #38556, #38732 ) ;
#13722=CARTESIAN_POINT ( 'NONE',  ( 789.9999999999992042, 205.0000000000000568, -329.9999999999999432 ) ) ;
#13727=DIRECTION ( 'NONE',  ( 0.000000000000000000, 0.000000000000000000, -1.000000000000000000 ) ) ;
#13729=VERTEX_POINT ( 'NONE', #23632 ) ;
#13746=AXIS2_PLACEMENT_3D ( 'NONE', #42113, #28019, #13263 ) ;
#13784=FACE_OUTER_BOUND ( 'NONE', #11618, .T. ) ;
#13793=CARTESIAN_POINT ( 'NONE',  ( -180.7583438952258916, 294.6698570112193920, -244.9999999999999716 ) ) ;
#13840=CARTESIAN_POINT ( 'NONE',  ( 200.7583438952259485, 394.6698570112193920, -274.9999999999999432 ) ) ;
#13877=CARTESIAN_POINT ( 'NONE',  ( 1238.921997096861332, 579.9999999999998863, -360.0000000000000000 ) ) ;
#13931=CARTESIAN_POINT ( 'NONE',  ( 794.9999999999993179, 205.0000000000000568, -255.0000000000000000 ) ) ;
#13963=DIRECTION ( 'NONE',  ( 1.000000000000000000, 0.000000000000000000, -0.000000000000000000 ) ) ;
#13990=ADVANCED_FACE ( 'NONE', ( #1386 ), #1603, .F. ) ;
#14008=ORIENTED_EDGE ( 'NONE', *, *, #28981, .T. ) ;
#14021=DIRECTION ( 'NONE',  ( 0.000000000000000000, 0.000000000000000000, -1.000000000000000000 ) ) ;
#14032=CARTESIAN_POINT ( 'NONE',  ( 794.9999999999993179, 205.0000000000000568, -255.0000000000000000 ) ) ;
#14103=VERTEX_POINT ( 'NONE', #17870 ) ;
#14134=DIRECTION ( 'NONE',  ( -5.551115123125783688E-16, 1.000000000000000000, 0.000000000000000000 ) ) ;
#14204=ORIENTED_EDGE ( 'NONE', *, *, #18199, .T. ) ;
#14216=EDGE_CURVE ( 'NONE', #26065, #45022, #44800, .T. ) ;
#14225=PLANE ( 'NONE',  #15167 ) ;
#14244=ADVANCED_FACE ( 'NONE', ( #16378 ), #37854, .F. ) ;
#14245=CARTESIAN_POINT ( 'NONE',  ( 200.7583438952258348, 240.0000000000006253, -244.9999999999999716 ) ) ;
#14254=EDGE_CURVE ( 'NONE', #41324, #38502, #44099, .T. ) ;
#14322=ORIENTED_EDGE ( 'NONE', *, *, #33474, .T. ) ;
#14363=CARTESIAN_POINT ( 'NONE',  ( -789.9999999999992042, 205.0000000000000568, -319.9999999999999432 ) ) ;
#14366=CARTESIAN_POINT ( 'NONE',  ( -789.9999999999992042, 205.0000000000000568, -360.0000000000000000 ) ) ;
#14388=CARTESIAN_POINT ( 'NONE',  ( 879.9999999999992042, 430.0000000000002842, -320.0000000000000568 ) ) ;
#14403=VECTOR ( 'NONE', #35136, 1000.000000000000000 ) ;
#14437=ADVANCED_BREP_SHAPE_REPRESENTATION ( '', ( #17465, #26858 ), #41617 ) ;
#14502=DIRECTION ( 'NONE',  ( -1.000000000000000000, 0.000000000000000000, 0.000000000000000000 ) ) ;
#14507=PLANE ( 'NONE',  #17974 ) ;
#14549=ADVANCED_FACE ( 'NONE', ( #21669 ), #13604, .F. ) ;
#14579=EDGE_CURVE ( 'NONE', #22309, #27668, #4803, .T. ) ;
#14610=FACE_OUTER_BOUND ( 'NONE', #6674, .T. ) ;
#14612=CARTESIAN_POINT ( 'NONE',  ( 1238.921997096861332, 430.0000000000002842, -320.0000000000000568 ) ) ;
#14656=DIRECTION ( 'NONE',  ( -0.000000000000000000, -0.000000000000000000, -1.000000000000000000 ) ) ;
#14713=DIRECTION ( 'NONE',  ( -1.000000000000000000, 0.000000000000000000, 0.000000000000000000 ) ) ;
#14716=EDGE_CURVE ( 'NONE', #45077, #33694, #40140, .T. ) ;
#14762=CARTESIAN_POINT ( 'NONE',  ( -829.9999999999992042, 290.0000000000001137, -244.9999999999999716 ) ) ;
#14809=CARTESIAN_POINT ( 'NONE',  ( 1238.921997096861332, 240.0000000000000568, -244.9999999999999716 ) ) ;
#14831=EDGE_CURVE ( 'NONE', #22309, #35390, #15221, .T. ) ;
#14861=EDGE_LOOP ( 'NONE', ( #1700, #28992, #22479, #8601 ) ) ;
#14865=ORIENTED_EDGE ( 'NONE', *, *, #9182, .F. ) ;
#14928=DIRECTION ( 'NONE',  ( -0.000000000000000000, 1.000000000000000000, -0.000000000000000000 ) ) ;
#14974=DIRECTION ( 'NONE',  ( 0.000000000000000000, 0.000000000000000000, -1.000000000000000000 ) ) ;
#14994=LINE ( 'NONE', #3691, #23238 ) ;
#15072=VECTOR ( 'NONE', #30913, 1000.000000000000000 ) ;
#15076=ORIENTED_EDGE ( 'NONE', *, *, #38818, .T. ) ;
#15112=EDGE_CURVE ( 'NONE', #15121, #22938, #13329, .T. ) ;
#15121=VERTEX_POINT ( 'NONE', #34336 ) ;
#15122=ADVANCED_FACE ( 'NONE', ( #20020 ), #23696, .F. ) ;
#15141=EDGE_CURVE ( 'NONE', #23098, #22342, #27815, .T. ) ;
#15157=CARTESIAN_POINT ( 'NONE',  ( 769.9999999999992042, 205.0000000000000568, -339.9999999999999432 ) ) ;
#15167=AXIS2_PLACEMENT_3D ( 'NONE', #18609, #7531, #25757 ) ;
#15184=AXIS2_PLACEMENT_3D ( 'NONE', #20150, #9540, #37710 ) ;
#15219=DIRECTION ( 'NONE',  ( 0.000000000000000000, 0.000000000000000000, 1.000000000000000000 ) ) ;
#15221=LINE ( 'NONE', #1552, #32237 ) ;
#15274=AXIS2_PLACEMENT_3D ( 'NONE', #1337, #25125, #15442 ) ;
#15309=VECTOR ( 'NONE', #29878, 1000.000000000000000 ) ;
#15323=FACE_OUTER_BOUND ( 'NONE', #28244, .T. ) ;
#15354=ORIENTED_EDGE ( 'NONE', *, *, #23000, .F. ) ;
#15361=ORIENTED_EDGE ( 'NONE', *, *, #24394, .T. ) ;
#15379=CARTESIAN_POINT ( 'NONE',  ( 1238.921997096861332, 430.0000000000002842, -244.9999999999999716 ) ) ;
#15385=DIRECTION ( 'NONE',  ( -0.000000000000000000, 1.000000000000000000, -0.000000000000000000 ) ) ;
#15399=CARTESIAN_POINT ( 'NONE',  ( 794.9999999999993179, 205.0000000000000568, -255.0000000000000000 ) ) ;
#15402=EDGE_CURVE ( 'NONE', #32155, #39971, #6842, .T. ) ;
#15409=ORIENTED_EDGE ( 'NONE', *, *, #41940, .T. ) ;
#15417=ORIENTED_EDGE ( 'NONE', *, *, #40798, .T. ) ;
#15425=ORIENTED_EDGE ( 'NONE', *, *, #30524, .F. ) ;
#15436=DIRECTION ( 'NONE',  ( -0.000000000000000000, -0.000000000000000000, 1.000000000000000000 ) ) ;
#15439=CIRCLE ( 'NONE', #41241, 10.00000000000006395 ) ;
#15442=DIRECTION ( 'NONE',  ( 0.000000000000000000, 0.000000000000000000, 1.000000000000000000 ) ) ;
#15457=ORIENTED_EDGE ( 'NONE', *, *, #43836, .F. ) ;
#15487=ORIENTED_EDGE ( 'NONE', *, *, #32318, .T. ) ;
#15490=DIRECTION ( 'NONE',  ( -1.000000000000000000, 0.000000000000000000, 0.000000000000000000 ) ) ;
#15491=CARTESIAN_POINT ( 'NONE',  ( -769.9999999999992042, 240.0000000000000853, -360.0000000000000000 ) ) ;
#15507=DIRECTION ( 'NONE',  ( -1.000000000000000000, -0.000000000000000000, -0.000000000000000000 ) ) ;
#15509=CARTESIAN_POINT ( 'NONE',  ( 190.7583438952259485, 394.6698570112193920, -274.9999999999999432 ) ) ;
#15552=CARTESIAN_POINT ( 'NONE',  ( -180.7583438952260622, 240.0000000000012506, -244.9999999999999716 ) ) ;
#15594=CARTESIAN_POINT ( 'NONE',  ( 794.9999999999993179, 205.0000000000000568, -235.0000000000000000 ) ) ;
#15601=CARTESIAN_POINT ( 'NONE',  ( -789.9999999999992042, 240.0000000000000568, -319.9999999999999432 ) ) ;
#15621=CIRCLE ( 'NONE', #13420, 10.00000000000000888 ) ;
#15650=DIRECTION ( 'NONE',  ( -1.000000000000000000, -0.000000000000000000, -0.000000000000000000 ) ) ;
#15736=DIRECTION ( 'NONE',  ( -1.000000000000000000, -0.000000000000000000, -0.000000000000000000 ) ) ;
#15758=ORIENTED_EDGE ( 'NONE', *, *, #35167, .T. ) ;
#15767=CARTESIAN_POINT ( 'NONE',  ( 794.9999999999993179, 240.0000000000000853, -275.0000000000000000 ) ) ;
#15811=FACE_OUTER_BOUND ( 'NONE', #13161, .T. ) ;
#15835=CARTESIAN_POINT ( 'NONE',  ( 355.8971257818259915, 290.0000000000001137, -244.9999999999999716 ) ) ;
#15847=AXIS2_PLACEMENT_3D ( 'NONE', #22589, #1785, #2027 ) ;
#15855=ORIENTED_EDGE ( 'NONE', *, *, #8274, .T. ) ;
#15857=VERTEX_POINT ( 'NONE', #25079 ) ;
#15872=DIRECTION ( 'NONE',  ( -0.000000000000000000, -4.857225732735055920E-15, 1.000000000000000000 ) ) ;
#15873=LINE ( 'NONE', #16563, #18959 ) ;
#15899=PLANE ( 'NONE',  #36598 ) ;
#15944=ADVANCED_FACE ( 'NONE', ( #42866 ), #11906, .T. ) ;
#16026=DIRECTION ( 'NONE',  ( 1.000000000000000000, 0.000000000000000000, 0.000000000000000000 ) ) ;
#16027=ORIENTED_EDGE ( 'NONE', *, *, #30039, .T. ) ;
#16047=CARTESIAN_POINT ( 'NONE',  ( 829.9999999999992042, 529.9999999999997726, -360.0000000000000000 ) ) ;
#16053=CARTESIAN_POINT ( 'NONE',  ( -115.7583438952258774, -600.0000000000000000, -244.9999999999999716 ) ) ;
#16077=DIRECTION ( 'NONE',  ( -1.000000000000000000, 0.000000000000000000, -0.000000000000000000 ) ) ;
#16086=EDGE_LOOP ( 'NONE', ( #8871, #42059, #21319, #33035 ) ) ;
#16106=CARTESIAN_POINT ( 'NONE',  ( -769.9999999999992042, 240.0000000000000568, -319.9999999999999432 ) ) ;
#16247=ORIENTED_EDGE ( 'NONE', *, *, #22162, .F. ) ;
#16249=ADVANCED_FACE ( 'NONE', ( #2403 ), #23421, .F. ) ;
#16254=EDGE_LOOP ( 'NONE', ( #29574, #31935, #32104, #8665, #25098, #15425, #37730, #1992, #28012, #40432, #29879, #12428, #29715, #20032, #1596, #36770 ) ) ;
#16267=ORIENTED_EDGE ( 'NONE', *, *, #11140, .T. ) ;
#16282=CARTESIAN_POINT ( 'NONE',  ( 769.9999999999992042, 205.0000000000000568, -350.0000000000000000 ) ) ;
#16283=CARTESIAN_POINT ( 'NONE',  ( 115.7583438952258774, 290.0000000000001705, -244.9999999999999716 ) ) ;
#16311=ORIENTED_EDGE ( 'NONE', *, *, #42547, .T. ) ;
#16329=DIRECTION ( 'NONE',  ( 8.326672684688676025E-16, 1.000000000000000000, -0.000000000000000000 ) ) ;
#16378=FACE_OUTER_BOUND ( 'NONE', #8920, .T. ) ;
#16382=VERTEX_POINT ( 'NONE', #38915 ) ;
#16394=AXIS2_PLACEMENT_3D ( 'NONE', #5037, #19129, #43383 ) ;
#16399=DIRECTION ( 'NONE',  ( 0.000000000000000000, 0.000000000000000000, -1.000000000000000000 ) ) ;
#16424=ADVANCED_FACE ( 'NONE', ( #10035 ), #23866, .F. ) ;
#16470=CARTESIAN_POINT ( 'NONE',  ( -200.7583438952259201, 394.6698570112193920, -244.9999999999999716 ) ) ;
#16476=ORIENTED_EDGE ( 'NONE', *, *, #38309, .F. ) ;
#16492=CARTESIAN_POINT ( 'NONE',  ( -879.9999999999992042, 240.0000000000000568, -244.9999999999999716 ) ) ;
#16504=DIRECTION ( 'NONE',  ( 0.000000000000000000, -1.000000000000000000, 0.000000000000000000 ) ) ;
#16520=EDGE_CURVE ( 'NONE', #19442, #30216, #3094, .T. ) ;
#16527=DIRECTION ( 'NONE',  ( -1.000000000000000000, -0.000000000000000000, -0.000000000000000000 ) ) ;
#16556=CIRCLE ( 'NONE', #25412, 50.00000000000004263 ) ;
#16562=DIRECTION ( 'NONE',  ( 0.000000000000000000, 0.000000000000000000, 1.000000000000000000 ) ) ;
#16563=CARTESIAN_POINT ( 'NONE',  ( 355.8971257818259915, 290.0000000000001137, -320.0000000000000568 ) ) ;
#16572=ORIENTED_EDGE ( 'NONE', *, *, #36240, .T. ) ;
#16574=AXIS2_PLACEMENT_3D ( 'NONE', #21055, #38387, #10662 ) ;
#16595=DIRECTION ( 'NONE',  ( 0.000000000000000000, 0.000000000000000000, 1.000000000000000000 ) ) ;
#16649=AXIS2_PLACEMENT_3D ( 'NONE', #31469, #29546, #24759 ) ;
#16712=EDGE_LOOP ( 'NONE', ( #3014, #32456, #32513, #1607 ) ) ;
#16729=ORIENTED_EDGE ( 'NONE', *, *, #21338, .F. ) ;
#16733=EDGE_LOOP ( 'NONE', ( #1145, #35864, #35603, #4955 ) ) ;
#16756=VECTOR ( 'NONE', #18615, 1000.000000000000000 ) ;
#16765=ORIENTED_EDGE ( 'NONE', *, *, #13105, .T. ) ;
#16779=EDGE_CURVE ( 'NONE', #45456, #2619, #8171, .T. ) ;
#16782=VERTEX_POINT ( 'NONE', #18113 ) ;
#16789=PLANE ( 'NONE',  #44657 ) ;
#16800=DIRECTION ( 'NONE',  ( -0.000000000000000000, -0.000000000000000000, 1.000000000000000000 ) ) ;
#16970=CARTESIAN_POINT ( 'NONE',  ( -789.9999999999992042, 205.0000000000000568, -339.9999999999999432 ) ) ;
#16984=FACE_OUTER_BOUND ( 'NONE', #24536, .T. ) ;
#16988=EDGE_LOOP ( 'NONE', ( #22738, #43009 ) ) ;
#16995=ORIENTED_EDGE ( 'NONE', *, *, #20200, .F. ) ;
#17015=DIRECTION ( 'NONE',  ( -0.000000000000000000, -0.000000000000000000, 1.000000000000000000 ) ) ;
#17048=CARTESIAN_POINT ( 'NONE',  ( 789.9999999999992042, 205.0000000000000568, -319.9999999999999432 ) ) ;
#17157=VECTOR ( 'NONE', #36440, 1000.000000000000000 ) ;
#17159=LINE ( 'NONE', #45341, #38211 ) ;
#17173=LINE ( 'NONE', #41896, #6616 ) ;
#17191=CARTESIAN_POINT ( 'NONE',  ( -769.9999999999992042, 205.0000000000000568, -319.9999999999999432 ) ) ;
#17202=DIRECTION ( 'NONE',  ( 1.000000000000000000, -0.000000000000000000, -0.000000000000000000 ) ) ;
#17206=VERTEX_POINT ( 'NONE', #27076 ) ;
#17212=ORIENTED_EDGE ( 'NONE', *, *, #689, .T. ) ;
#17246=EDGE_CURVE ( 'NONE', #38502, #31293, #22690, .T. ) ;
#17307=CARTESIAN_POINT ( 'NONE',  ( 789.9999999999992042, 240.0000000000000568, -319.9999999999999432 ) ) ;
#17312=CARTESIAN_POINT ( 'NONE',  ( 769.9999999999992042, 205.0000000000000568, -329.9999999999999432 ) ) ;
#17330=PLANE ( 'NONE',  #30818 ) ;
#17331=ORIENTED_EDGE ( 'NONE', *, *, #36744, .T. ) ;
#17353=ORIENTED_EDGE ( 'NONE', *, *, #4112, .F. ) ;
#17372=LINE ( 'NONE', #18060, #6546 ) ;
#17385=PLANE ( 'NONE',  #16649 ) ;
#17406=VECTOR ( 'NONE', #15385, 1000.000000000000000 ) ;
#17416=CIRCLE ( 'NONE', #43222, 10.00000000000006395 ) ;
#17425=FACE_OUTER_BOUND ( 'NONE', #5011, .T. ) ;
#17442=VECTOR ( 'NONE', #21391, 1000.000000000000000 ) ;
#17447=DIRECTION ( 'NONE',  ( -0.000000000000000000, 1.000000000000000000, 0.000000000000000000 ) ) ;
#17465=MANIFOLD_SOLID_BREP ( 'Fillet1', #37218 ) ;
#17474=CARTESIAN_POINT ( 'NONE',  ( 829.9999999999992042, 529.9999999999997726, -320.0000000000000000 ) ) ;
#17490=DIRECTION ( 'NONE',  ( -1.000000000000000000, -0.000000000000000000, -0.000000000000000000 ) ) ;
#17491=CIRCLE ( 'NONE', #31484, 50.00000000000004263 ) ;
#17524=ORIENTED_EDGE ( 'NONE', *, *, #6286, .F. ) ;
#17569=EDGE_CURVE ( 'NONE', #32576, #8421, #15621, .T. ) ;
#17604=DIRECTION ( 'NONE',  ( 0.000000000000000000, -1.000000000000000000, 0.000000000000000000 ) ) ;
#17628=EDGE_LOOP ( 'NONE', ( #42680, #20843, #15409, #29655 ) ) ;
#17648=DIRECTION ( 'NONE',  ( 5.551115123125783688E-16, 1.000000000000000000, 0.000000000000000000 ) ) ;
#17650=ORIENTED_EDGE ( 'NONE', *, *, #22976, .F. ) ;
#17679=CARTESIAN_POINT ( 'NONE',  ( 355.8971257818259915, 290.0000000000001137, -244.9999999999999716 ) ) ;
#17684=EDGE_CURVE ( 'NONE', #27240, #22001, #11930, .T. ) ;
#17712=CARTESIAN_POINT ( 'NONE',  ( 190.7583438952259485, 394.6698570112193920, -274.9999999999999432 ) ) ;
#17717=CARTESIAN_POINT ( 'NONE',  ( 1238.921997096861332, 240.0000000000000853, -360.0000000000000000 ) ) ;
#17723=EDGE_CURVE ( 'NONE', #32851, #66, #32132, .T. ) ;
#17743=ORIENTED_EDGE ( 'NONE', *, *, #45522, .T. ) ;
#17808=LINE ( 'NONE', #42739, #12268 ) ;
#17870=CARTESIAN_POINT ( 'NONE',  ( 829.9999999999992042, 290.0000000000001137, -320.0000000000000568 ) ) ;
#17956=CARTESIAN_POINT ( 'NONE',  ( 789.9999999999992042, 205.0000000000000568, -319.9999999999999432 ) ) ;
#17974=AXIS2_PLACEMENT_3D ( 'NONE', #28585, #16077, #27162 ) ;
#17990=CARTESIAN_POINT ( 'NONE',  ( 784.9999999999992042, 205.0000000000000568, -255.0000000000000000 ) ) ;
#18056=AXIS2_PLACEMENT_3D ( 'NONE', #36285, #4871, #18739 ) ;
#18060=CARTESIAN_POINT ( 'NONE',  ( -200.7583438952258348, 239.9999999999992326, -244.9999999999999716 ) ) ;
#18071=VECTOR ( 'NONE', #18638, 1000.000000000000000 ) ;
#18090=VERTEX_POINT ( 'NONE', #29798 ) ;
#18101=PLANE ( 'NONE',  #8644 ) ;
#18106=ORIENTED_EDGE ( 'NONE', *, *, #6607, .F. ) ;
#18113=CARTESIAN_POINT ( 'NONE',  ( -829.9999999999994316, 579.9999999999998863, -360.0000000000000000 ) ) ;
#18155=CIRCLE ( 'NONE', #29189, 10.00000000000000888 ) ;
#18165=ORIENTED_EDGE ( 'NONE', *, *, #14254, .F. ) ;
#18198=ORIENTED_EDGE ( 'NONE', *, *, #15402, .T. ) ;
#18199=EDGE_CURVE ( 'NONE', #39971, #11672, #44110, .T. ) ;
#18218=VECTOR ( 'NONE', #19335, 1000.000000000000000 ) ;
#18231=ADVANCED_FACE ( 'NONE', ( #4086 ), #27248, .F. ) ;
#18288=ORIENTED_EDGE ( 'NONE', *, *, #15112, .F. ) ;
#18355=PLANE ( 'NONE',  #10629 ) ;
#18388=CARTESIAN_POINT ( 'NONE',  ( 794.9999999999993179, 205.0000000000000568, -255.0000000000000000 ) ) ;
#18532=EDGE_CURVE ( 'NONE', #22342, #23098, #38746, .T. ) ;
#18559=EDGE_CURVE ( 'NONE', #34504, #36537, #4746, .T. ) ;
#18595=ORIENTED_EDGE ( 'NONE', *, *, #41940, .F. ) ;
#18609=CARTESIAN_POINT ( 'NONE',  ( 1238.921997096861332, 240.0000000000000853, -360.0000000000000000 ) ) ;
#18615=DIRECTION ( 'NONE',  ( -0.000000000000000000, -0.000000000000000000, 1.000000000000000000 ) ) ;
#18638=DIRECTION ( 'NONE',  ( -0.000000000000000000, -0.000000000000000000, 1.000000000000000000 ) ) ;
#18651=VERTEX_POINT ( 'NONE', #32940 ) ;
#18669=DIRECTION ( 'NONE',  ( -1.000000000000000000, 0.000000000000000000, 0.000000000000000000 ) ) ;
#18672=DIRECTION ( 'NONE',  ( 0.000000000000000000, 0.000000000000000000, 1.000000000000000000 ) ) ;
#18694=CARTESIAN_POINT ( 'NONE',  ( 1238.921997096861332, 430.0000000000002842, -320.0000000000000568 ) ) ;
#18710=AXIS2_PLACEMENT_3D ( 'NONE', #12422, #34103, #29971 ) ;
#18716=EDGE_LOOP ( 'NONE', ( #26077, #21774, #44804, #6999, #539 ) ) ;
#18724=EDGE_LOOP ( 'NONE', ( #8540, #8368, #25902, #18106 ) ) ;
#18732=EDGE_CURVE ( 'NONE', #11266, #31293, #829, .T. ) ;
#18739=DIRECTION ( 'NONE',  ( 1.000000000000000000, 0.000000000000000000, 0.000000000000000000 ) ) ;
#18760=DIRECTION ( 'NONE',  ( -0.000000000000000000, -6.938893903907241197E-16, 1.000000000000000000 ) ) ;
#18767=AXIS2_PLACEMENT_3D ( 'NONE', #33843, #41461, #30370 ) ;
#18807=ADVANCED_FACE ( 'NONE', ( #40541 ), #26214, .F. ) ;
#18871=CARTESIAN_POINT ( 'NONE',  ( 879.9999999999992042, 529.9999999999997726, -244.9999999999999716 ) ) ;
#18929=CIRCLE ( 'NONE', #9354, 10.00000000000000888 ) ;
#18940=ORIENTED_EDGE ( 'NONE', *, *, #23484, .F. ) ;
#18941=VERTEX_POINT ( 'NONE', #31440 ) ;
#18959=VECTOR ( 'NONE', #44745, 1000.000000000000000 ) ;
#18973=FACE_OUTER_BOUND ( 'NONE', #44593, .T. ) ;
#19019=APPLICATION_CONTEXT ( 'automotive_design' ) ;
#19054=AXIS2_PLACEMENT_3D ( 'NONE', #14032, #44986, #13342 ) ;
#19074=CARTESIAN_POINT ( 'NONE',  ( 784.9999999999992042, 239.9999999999998863, -235.0000000000000000 ) ) ;
#19094=LINE ( 'NONE', #8703, #6282 ) ;
#19122=AXIS2_PLACEMENT_3D ( 'NONE', #21739, #32830, #33067 ) ;
#19129=DIRECTION ( 'NONE',  ( -1.000000000000000000, -5.551115123125783688E-16, 0.000000000000000000 ) ) ;
#19166=EDGE_LOOP ( 'NONE', ( #9498, #3754, #11831, #13009 ) ) ;
#19248=ORIENTED_EDGE ( 'NONE', *, *, #12079, .T. ) ;
#19302=DIRECTION ( 'NONE',  ( 0.000000000000000000, 3.700743415417198493E-16, -1.000000000000000000 ) ) ;
#19305=ORIENTED_EDGE ( 'NONE', *, *, #40995, .F. ) ;
#19317=EDGE_CURVE ( 'NONE', #45456, #6536, #9953, .T. ) ;
#19335=DIRECTION ( 'NONE',  ( -0.000000000000000000, -0.000000000000000000, 1.000000000000000000 ) ) ;
#19342=AXIS2_PLACEMENT_3D ( 'NONE', #39432, #25090, #21632 ) ;
#19358=ORIENTED_EDGE ( 'NONE', *, *, #39941, .F. ) ;
#19361=VECTOR ( 'NONE', #37350, 1000.000000000000000 ) ;
#19366=ORIENTED_EDGE ( 'NONE', *, *, #43078, .F. ) ;
#19367=EDGE_CURVE ( 'NONE', #33185, #18651, #18155, .T. ) ;
#19375=ORIENTED_EDGE ( 'NONE', *, *, #38536, .T. ) ;
#19442=VERTEX_POINT ( 'NONE', #35028 ) ;
#19450=AXIS2_PLACEMENT_3D ( 'NONE', #37062, #12589, #26667 ) ;
#19465=VECTOR ( 'NONE', #33313, 1000.000000000000000 ) ;
#19474=CARTESIAN_POINT ( 'NONE',  ( 769.9999999999992042, 205.0000000000000568, -339.9999999999999432 ) ) ;
#19523=CARTESIAN_POINT ( 'NONE',  ( 355.8971257818259915, 290.0000000000001137, -244.9999999999999716 ) ) ;
#19567=VECTOR ( 'NONE', #26553, 1000.000000000000000 ) ;
#19615=DIRECTION ( 'NONE',  ( 0.000000000000000000, -1.000000000000000000, 0.000000000000000000 ) ) ;
#19641=VECTOR ( 'NONE', #24213, 1000.000000000000000 ) ;
#19660=VECTOR ( 'NONE', #19846, 1000.000000000000000 ) ;
#19729=CARTESIAN_POINT ( 'NONE',  ( -789.9999999999992042, 205.0000000000000568, -339.9999999999999432 ) ) ;
#19732=LINE ( 'NONE', #20410, #412 ) ;
#19734=VERTEX_POINT ( 'NONE', #6166 ) ;
#19810=VERTEX_POINT ( 'NONE', #20256 ) ;
#19846=DIRECTION ( 'NONE',  ( -0.000000000000000000, 1.000000000000000000, -0.000000000000000000 ) ) ;
#19895=ADVANCED_FACE ( 'NONE', ( #7333 ), #38742, .F. ) ;
#19941=DIRECTION ( 'NONE',  ( -0.000000000000000000, -0.000000000000000000, 1.000000000000000000 ) ) ;
#19958=DIRECTION ( 'NONE',  ( 1.000000000000000000, 0.000000000000000000, 0.000000000000000000 ) ) ;
#19963=LINE ( 'NONE', #43746, #24809 ) ;
#20020=FACE_OUTER_BOUND ( 'NONE', #45347, .T. ) ;
#20032=ORIENTED_EDGE ( 'NONE', *, *, #17246, .F. ) ;
#20042=FACE_OUTER_BOUND ( 'NONE', #18716, .T. ) ;
#20084=CARTESIAN_POINT ( 'NONE',  ( -200.7583438952258916, 294.6698570112193920, -274.9999999999999432 ) ) ;
#20134=CARTESIAN_POINT ( 'NONE',  ( 784.9999999999992042, 239.9999999999998863, -235.0000000000000000 ) ) ;
#20150=CARTESIAN_POINT ( 'NONE',  ( -190.7583438952258916, 294.6698570112193920, -274.9999999999999432 ) ) ;
#20152=ORIENTED_EDGE ( 'NONE', *, *, #4945, .T. ) ;
#20163=VECTOR ( 'NONE', #45403, 1000.000000000000000 ) ;
#20183=ORIENTED_EDGE ( 'NONE', *, *, #23550, .F. ) ;
#20200=EDGE_CURVE ( 'NONE', #43685, #16782, #16556, .T. ) ;
#20210=CARTESIAN_POINT ( 'NONE',  ( 115.7583438952258774, 290.0000000000001137, -320.0000000000000568 ) ) ;
#20235=LINE ( 'NONE', #34323, #26225 ) ;
#20256=CARTESIAN_POINT ( 'NONE',  ( -879.9999999999992042, 430.0000000000002842, -244.9999999999999716 ) ) ;
#20271=CARTESIAN_POINT ( 'NONE',  ( 784.9999999999992042, 205.0000000000000568, -265.0000000000000000 ) ) ;
#20327=ORIENTED_EDGE ( 'NONE', *, *, #30611, .F. ) ;
#20350=AXIS2_PLACEMENT_3D ( 'NONE', #16970, #13963, #27579 ) ;
#20360=SHAPE_REPRESENTATION ( 'Moving Blade Support Base', ( #26858 ), #41617 ) ;
#20374=CARTESIAN_POINT ( 'NONE',  ( 784.9999999999992042, 205.0000000000000568, -235.0000000000000284 ) ) ;
#20380=PLANE ( 'NONE',  #21792 ) ;
#20388=AXIS2_PLACEMENT_3D ( 'NONE', #29306, #18669, #15219 ) ;
#20390=FACE_OUTER_BOUND ( 'NONE', #11611, .T. ) ;
#20410=CARTESIAN_POINT ( 'NONE',  ( 784.9999999999992042, 205.0000000000000568, -235.0000000000000000 ) ) ;
#20454=CARTESIAN_POINT ( 'NONE',  ( -829.9999999999992042, 430.0000000000002842, -244.9999999999995168 ) ) ;
#20468=EDGE_CURVE ( 'NONE', #30216, #11266, #6217, .T. ) ;
#20486=DIRECTION ( 'NONE',  ( -0.000000000000000000, 1.000000000000000000, -0.000000000000000000 ) ) ;
#20497=ORIENTED_EDGE ( 'NONE', *, *, #26039, .F. ) ;
#20500=VECTOR ( 'NONE', #28467, 1000.000000000000000 ) ;
#20512=ORIENTED_EDGE ( 'NONE', *, *, #21338, .T. ) ;
#20527=ORIENTED_EDGE ( 'NONE', *, *, #35398, .F. ) ;
#20566=CARTESIAN_POINT ( 'NONE',  ( 829.9999999999992042, -600.0000000000000000, -244.9999999999999716 ) ) ;
#20567=ORIENTED_EDGE ( 'NONE', *, *, #37668, .T. ) ;
#20586=VECTOR ( 'NONE', #34645, 1000.000000000000000 ) ;
#20606=CARTESIAN_POINT ( 'NONE',  ( 769.9999999999992042, 205.0000000000000568, -319.9999999999999432 ) ) ;
#20622=ORIENTED_EDGE ( 'NONE', *, *, #38917, .T. ) ;
#20633=DIRECTION ( 'NONE',  ( 0.000000000000000000, 0.000000000000000000, 1.000000000000000000 ) ) ;
#20693=CARTESIAN_POINT ( 'NONE',  ( 794.9999999999993179, 205.0000000000000568, -235.0000000000000284 ) ) ;
#20695=EDGE_CURVE ( 'NONE', #44609, #9031, #41641, .T. ) ;
#20737=DIRECTION ( 'NONE',  ( -0.000000000000000000, 1.000000000000000000, -0.000000000000000000 ) ) ;
#20742=CARTESIAN_POINT ( 'NONE',  ( -829.9999999999994316, 579.9999999999998863, -320.0000000000000000 ) ) ;
#20825=FACE_OUTER_BOUND ( 'NONE', #20887, .T. ) ;
#20840=SHAPE_REPRESENTATION_RELATIONSHIP ( 'NONE' , 'NONE' ,  #20360, #14437 ) ;
#20843=ORIENTED_EDGE ( 'NONE', *, *, #43599, .F. ) ;
#20887=EDGE_LOOP ( 'NONE', ( #2035, #18288, #16267, #4731 ) ) ;
#20923=LINE ( 'NONE', #17717, #8328 ) ;
#20932=FACE_OUTER_BOUND ( 'NONE', #16733, .T. ) ;
#20935=ORIENTED_EDGE ( 'NONE', *, *, #30039, .F. ) ;
#20936=VECTOR ( 'NONE', #39361, 1000.000000000000000 ) ;
#20965=CARTESIAN_POINT ( 'NONE',  ( -190.7583438952259485, 290.0000000000001137, -274.9999999999999432 ) ) ;
#21055=CARTESIAN_POINT ( 'NONE',  ( 769.9999999999992042, 205.0000000000000568, -339.9999999999999432 ) ) ;
#21056=VECTOR ( 'NONE', #11251, 1000.000000000000000 ) ;
#21062=CIRCLE ( 'NONE', #15184, 10.00000000000000888 ) ;
#21071=DIRECTION ( 'NONE',  ( -1.000000000000000000, -0.000000000000000000, -0.000000000000000000 ) ) ;
#21084=ORIENTED_EDGE ( 'NONE', *, *, #35683, .T. ) ;
#21094=EDGE_LOOP ( 'NONE', ( #23456, #13256, #1876, #17524 ) ) ;
#21103=PRODUCT ( 'Moving Blade Support Base', 'Moving Blade Support Base', '', ( #11267 ) ) ;
#21106=FACE_OUTER_BOUND ( 'NONE', #8926, .T. ) ;
#21110=PLANE ( 'NONE',  #33485 ) ;
#21116=PLANE ( 'NONE',  #20350 ) ;
#21120=DIRECTION ( 'NONE',  ( -8.326672684688676025E-16, 1.000000000000000000, 0.000000000000000000 ) ) ;
#21150=VERTEX_POINT ( 'NONE', #32205 ) ;
#21164=AXIS2_PLACEMENT_3D ( 'NONE', #27741, #23579, #37684 ) ;
#21172=AXIS2_PLACEMENT_3D ( 'NONE', #37570, #26944, #16562 ) ;
#21183=CARTESIAN_POINT ( 'NONE',  ( 769.9999999999992042, 205.0000000000000568, -339.9999999999999432 ) ) ;
#21280=CARTESIAN_POINT ( 'NONE',  ( 190.7583438952258916, 294.6698570112193920, -274.9999999999999432 ) ) ;
#21319=ORIENTED_EDGE ( 'NONE', *, *, #11931, .F. ) ;
#21338=EDGE_CURVE ( 'NONE', #13729, #39585, #40198, .T. ) ;
#21339=DIRECTION ( 'NONE',  ( 0.000000000000000000, -0.000000000000000000, -1.000000000000000000 ) ) ;
#21377=APPLICATION_CONTEXT ( 'automotive_design' ) ;
#21391=DIRECTION ( 'NONE',  ( 5.551115123125783688E-16, 1.000000000000000000, -0.000000000000000000 ) ) ;
#21509=PLANE ( 'NONE',  #3605 ) ;
#21532=VERTEX_POINT ( 'NONE', #39611 ) ;
#21541=ORIENTED_EDGE ( 'NONE', *, *, #36744, .F. ) ;
#21551=ORIENTED_EDGE ( 'NONE', *, *, #3479, .T. ) ;
#21553=AXIS2_PLACEMENT_3D ( 'NONE', #10715, #10477, #21339 ) ;
#21557=DIRECTION ( 'NONE',  ( -1.000000000000000000, 0.000000000000000000, 0.000000000000000000 ) ) ;
#21564=FACE_OUTER_BOUND ( 'NONE', #35623, .T. ) ;
#21589=ORIENTED_EDGE ( 'NONE', *, *, #12079, .F. ) ;
#21600=ORIENTED_EDGE ( 'NONE', *, *, #13183, .T. ) ;
#21619=DIRECTION ( 'NONE',  ( -1.000000000000000000, 0.000000000000000000, 0.000000000000000000 ) ) ;
#21632=DIRECTION ( 'NONE',  ( 0.000000000000000000, 0.000000000000000000, -1.000000000000000000 ) ) ;
#21654=SHAPE_DEFINITION_REPRESENTATION ( #42502, #20360 ) ;
#21669=FACE_OUTER_BOUND ( 'NONE', #30799, .T. ) ;
#21696=ORIENTED_EDGE ( 'NONE', *, *, #17723, .F. ) ;
#21739=CARTESIAN_POINT ( 'NONE',  ( -769.9999999999992042, 205.0000000000000568, -339.9999999999999432 ) ) ;
#21774=ORIENTED_EDGE ( 'NONE', *, *, #8131, .F. ) ;
#21792=AXIS2_PLACEMENT_3D ( 'NONE', #20606, #6527, #41411 ) ;
#21837=ORIENTED_EDGE ( 'NONE', *, *, #30318, .T. ) ;
#21867=ADVANCED_FACE ( 'NONE', ( #22767 ), #40775, .T. ) ;
#21888=VECTOR ( 'NONE', #37571, 1000.000000000000000 ) ;
#21916=VERTEX_POINT ( 'NONE', #24570 ) ;
#21934=EDGE_LOOP ( 'NONE', ( #9569, #44604, #10445, #40787 ) ) ;
#21946=ADVANCED_FACE ( 'NONE', ( #31529 ), #13067, .T. ) ;
#22001=VERTEX_POINT ( 'NONE', #45394 ) ;
#22012=PLANE ( 'NONE',  #36582 ) ;
#22016=VERTEX_POINT ( 'NONE', #31061 ) ;
#22063=DIRECTION ( 'NONE',  ( 0.000000000000000000, 1.000000000000000000, 0.000000000000000000 ) ) ;
#22066=ADVANCED_FACE ( 'NONE', ( #41465, #16984 ), #23885, .T. ) ;
#22074=CARTESIAN_POINT ( 'NONE',  ( 789.9999999999992042, 240.0000000000000853, -360.0000000000000000 ) ) ;
#22094=LINE ( 'NONE', #4767, #21056 ) ;
#22125=FACE_OUTER_BOUND ( 'NONE', #26514, .T. ) ;
#22135=EDGE_CURVE ( 'NONE', #45115, #2619, #45631, .T. ) ;
#22146=ORIENTED_EDGE ( 'NONE', *, *, #28278, .T. ) ;
#22162=EDGE_CURVE ( 'NONE', #2619, #37165, #45412, .T. ) ;
#22173=LINE ( 'NONE', #15491, #44524 ) ;
#22192=DIRECTION ( 'NONE',  ( -0.000000000000000000, 1.000000000000000000, 0.000000000000000000 ) ) ;
#22212=ORIENTED_EDGE ( 'NONE', *, *, #26992, .T. ) ;
#22236=MECHANICAL_DESIGN_GEOMETRIC_PRESENTATION_REPRESENTATION('',(#42162),#2316);
#22240=LINE ( 'NONE', #15552, #20936 ) ;
#22256=ORIENTED_EDGE ( 'NONE', *, *, #45035, .T. ) ;
#22295=CARTESIAN_POINT ( 'NONE',  ( 794.9999999999993179, 239.9999999999998863, -235.0000000000000000 ) ) ;
#22309=VERTEX_POINT ( 'NONE', #20210 ) ;
#22342=VERTEX_POINT ( 'NONE', #25044 ) ;
#22358=ORIENTED_EDGE ( 'NONE', *, *, #25547, .F. ) ;
#22360=EDGE_CURVE ( 'NONE', #33022, #38320, #39153, .T. ) ;
#22413=CIRCLE ( 'NONE', #6933, 10.00000000000000888 ) ;
#22414=VECTOR ( 'NONE', #33606, 1000.000000000000000 ) ;
#22425=CARTESIAN_POINT ( 'NONE',  ( -879.9999999999992042, 240.0000000000000853, -360.0000000000000000 ) ) ;
#22479=ORIENTED_EDGE ( 'NONE', *, *, #36240, .F. ) ;
#22486=ORIENTED_EDGE ( 'NONE', *, *, #28278, .F. ) ;
#22530=FACE_OUTER_BOUND ( 'NONE', #289, .T. ) ;
#22571=LINE ( 'NONE', #8503, #12296 ) ;
#22589=CARTESIAN_POINT ( 'NONE',  ( 794.9999999999993179, 205.0000000000000568, -255.0000000000000000 ) ) ;
#22606=VERTEX_POINT ( 'NONE', #29207 ) ;
#22664=ORIENTED_EDGE ( 'NONE', *, *, #39050, .T. ) ;
#22690=LINE ( 'NONE', #36787, #40703 ) ;
#22702=EDGE_LOOP ( 'NONE', ( #16572, #27954, #22486, #19305, #3553, #31711, #36135, #25010, #904, #3384, #2374, #25845, #35930, #45125, #37859, #33471, #42569, #38240 ) ) ;
#22738=ORIENTED_EDGE ( 'NONE', *, *, #13412, .T. ) ;
#22767=FACE_OUTER_BOUND ( 'NONE', #16086, .T. ) ;
#22938=VERTEX_POINT ( 'NONE', #10217 ) ;
#22945=FACE_OUTER_BOUND ( 'NONE', #205, .T. ) ;
#22950=ORIENTED_EDGE ( 'NONE', *, *, #25197, .F. ) ;
#22966=CARTESIAN_POINT ( 'NONE',  ( 1238.921997096861332, 430.0000000000002842, -244.9999999999999716 ) ) ;
#22967=PLANE ( 'NONE',  #19450 ) ;
#22976=EDGE_CURVE ( 'NONE', #12562, #15121, #21062, .T. ) ;
#23000=EDGE_CURVE ( 'NONE', #24825, #40516, #44645, .T. ) ;
#23011=CARTESIAN_POINT ( 'NONE',  ( 769.9999999999992042, 205.0000000000000568, -360.0000000000000000 ) ) ;
#23017=ADVANCED_FACE ( 'NONE', ( #2601 ), #20380, .T. ) ;
#23098=VERTEX_POINT ( 'NONE', #45107 ) ;
#23150=ORIENTED_EDGE ( 'NONE', *, *, #19367, .F. ) ;
#23153=CARTESIAN_POINT ( 'NONE',  ( 0.000000000000000000, 0.000000000000000000, 0.000000000000000000 ) ) ;
#23168=VERTEX_POINT ( 'NONE', #23826 ) ;
#23172=ORIENTED_EDGE ( 'NONE', *, *, #34811, .T. ) ;
#23238=VECTOR ( 'NONE', #7849, 1000.000000000000000 ) ;
#23247=DIRECTION ( 'NONE',  ( 0.000000000000000000, 0.000000000000000000, -1.000000000000000000 ) ) ;
#23296=ORIENTED_EDGE ( 'NONE', *, *, #11651, .F. ) ;
#23302=DIRECTION ( 'NONE',  ( -1.000000000000000000, -0.000000000000000000, -0.000000000000000000 ) ) ;
#23321=DIRECTION ( 'NONE',  ( 0.000000000000000000, 0.000000000000000000, -1.000000000000000000 ) ) ;
#23387=VECTOR ( 'NONE', #23417, 1000.000000000000000 ) ;
#23417=DIRECTION ( 'NONE',  ( 0.000000000000000000, 0.000000000000000000, 1.000000000000000000 ) ) ;
#23421=PLANE ( 'NONE',  #28175 ) ;
#23456=ORIENTED_EDGE ( 'NONE', *, *, #34274, .F. ) ;
#23470=CARTESIAN_POINT ( 'NONE',  ( 200.7583438952258916, 294.6698570112193920, -274.9999999999999432 ) ) ;
#23480=CARTESIAN_POINT ( 'NONE',  ( 794.9999999999993179, 205.0000000000000568, -274.9999999999999432 ) ) ;
#23484=EDGE_CURVE ( 'NONE', #18090, #24825, #5593, .T. ) ;
#23517=ORIENTED_EDGE ( 'NONE', *, *, #44081, .F. ) ;
#23550=EDGE_CURVE ( 'NONE', #36814, #2255, #7838, .T. ) ;
#23560=EDGE_CURVE ( 'NONE', #34305, #2122, #17416, .T. ) ;
#23570=ORIENTED_EDGE ( 'NONE', *, *, #35112, .T. ) ;
#23579=DIRECTION ( 'NONE',  ( 0.000000000000000000, -1.000000000000000000, -0.000000000000000000 ) ) ;
#23594=CYLINDRICAL_SURFACE ( 'NONE', #43416, 9.999999999999980460 ) ;
#23598=DIRECTION ( 'NONE',  ( -1.000000000000000000, 0.000000000000000000, 0.000000000000000000 ) ) ;
#23632=CARTESIAN_POINT ( 'NONE',  ( 199.6009925648704098, 290.0000000000001137, -274.9999999999999432 ) ) ;
#23663=ORIENTED_EDGE ( 'NONE', *, *, #30014, .F. ) ;
#23696=CYLINDRICAL_SURFACE ( 'NONE', #1986, 10.00000000000000888 ) ;
#23702=DIRECTION ( 'NONE',  ( 0.000000000000000000, 0.000000000000000000, -1.000000000000000000 ) ) ;
#23787=ADVANCED_FACE ( 'NONE', ( #11220 ), #42638, .F. ) ;
#23826=CARTESIAN_POINT ( 'NONE',  ( -769.9999999999992042, 205.0000000000000568, -329.9999999999999432 ) ) ;
#23845=ORIENTED_EDGE ( 'NONE', *, *, #5113, .F. ) ;
#23847=ORIENTED_EDGE ( 'NONE', *, *, #29307, .F. ) ;
#23866=PLANE ( 'NONE',  #21553 ) ;
#23885=PLANE ( 'NONE',  #24681 ) ;
#24018=DIRECTION ( 'NONE',  ( -0.000000000000000000, 1.000000000000000000, 0.000000000000000000 ) ) ;
#24031=FACE_OUTER_BOUND ( 'NONE', #30915, .T. ) ;
#24062=DIRECTION ( 'NONE',  ( 0.000000000000000000, 0.000000000000000000, -1.000000000000000000 ) ) ;
#24089=CARTESIAN_POINT ( 'NONE',  ( -190.7583438952258916, 294.6698570112193920, -274.9999999999999432 ) ) ;
#24094=ORIENTED_EDGE ( 'NONE', *, *, #38114, .T. ) ;
#24098=CARTESIAN_POINT ( 'NONE',  ( -769.9999999999992042, 205.0000000000000568, -339.9999999999999432 ) ) ;
#24105=VECTOR ( 'NONE', #879, 1000.000000000000000 ) ;
#24130=ORIENTED_EDGE ( 'NONE', *, *, #44450, .F. ) ;
#24171=EDGE_CURVE ( 'NONE', #33185, #22001, #30809, .T. ) ;
#24213=DIRECTION ( 'NONE',  ( -0.000000000000000000, -0.000000000000000000, 1.000000000000000000 ) ) ;
#24309=( LENGTH_UNIT ( ) NAMED_UNIT ( * ) SI_UNIT ( .MILLI., .METRE. ) );
#24381=CARTESIAN_POINT ( 'NONE',  ( 200.7583438952259485, 394.6698570112193920, -274.9999999999999432 ) ) ;
#24394=EDGE_CURVE ( 'NONE', #13729, #22001, #17808, .T. ) ;
#24412=ORIENTED_EDGE ( 'NONE', *, *, #16520, .F. ) ;
#24413=EDGE_CURVE ( 'NONE', #44613, #36817, #25173, .T. ) ;
#24484=ORIENTED_EDGE ( 'NONE', *, *, #24171, .T. ) ;
#24501=LINE ( 'NONE', #20134, #14403 ) ;
#24528=CARTESIAN_POINT ( 'NONE',  ( 115.7583438952258774, 290.0000000000001705, -244.9999999999999716 ) ) ;
#24531=EDGE_LOOP ( 'NONE', ( #23845, #43413, #7373, #22212 ) ) ;
#24536=EDGE_LOOP ( 'NONE', ( #11336, #3595, #21541, #22358 ) ) ;
#24545=CARTESIAN_POINT ( 'NONE',  ( 784.9999999999992042, 205.0000000000000568, -255.0000000000000000 ) ) ;
#24555=LINE ( 'NONE', #38439, #29849 ) ;
#24570=CARTESIAN_POINT ( 'NONE',  ( -115.7583438952258774, 290.0000000000001137, -244.9999999999999716 ) ) ;
#24622=DIRECTION ( 'NONE',  ( -1.000000000000000000, -0.000000000000000000, -0.000000000000000000 ) ) ;
#24681=AXIS2_PLACEMENT_3D ( 'NONE', #10274, #38008, #30841 ) ;
#24737=DIRECTION ( 'NONE',  ( 1.000000000000000000, 0.000000000000000000, 0.000000000000000000 ) ) ;
#24759=DIRECTION ( 'NONE',  ( 8.326672684688676025E-16, 1.000000000000000000, 0.000000000000000000 ) ) ;
#24779=ORIENTED_EDGE ( 'NONE', *, *, #27519, .T. ) ;
#24809=VECTOR ( 'NONE', #1702, 1000.000000000000000 ) ;
#24825=VERTEX_POINT ( 'NONE', #37402 ) ;
#24839=VECTOR ( 'NONE', #19615, 1000.000000000000000 ) ;
#24841=DIRECTION ( 'NONE',  ( -0.000000000000000000, -0.000000000000000000, 1.000000000000000000 ) ) ;
#24875=ORIENTED_EDGE ( 'NONE', *, *, #11726, .T. ) ;
#24938=LINE ( 'NONE', #11091, #41174 ) ;
#24949=ORIENTED_EDGE ( 'NONE', *, *, #23560, .F. ) ;
#24954=CARTESIAN_POINT ( 'NONE',  ( 829.9999999999992042, 579.9999999999998863, -360.0000000000000000 ) ) ;
#24995=ORIENTED_EDGE ( 'NONE', *, *, #35398, .T. ) ;
#25010=ORIENTED_EDGE ( 'NONE', *, *, #2909, .F. ) ;
#25018=VERTEX_POINT ( 'NONE', #42014 ) ;
#25043=CIRCLE ( 'NONE', #44969, 10.00000000000000888 ) ;
#25044=CARTESIAN_POINT ( 'NONE',  ( 769.9999999999992042, 205.0000000000000568, -329.9999999999999432 ) ) ;
#25048=EDGE_LOOP ( 'NONE', ( #44978, #2797 ) ) ;
#25054=ORIENTED_EDGE ( 'NONE', *, *, #4027, .T. ) ;
#25063=ORIENTED_EDGE ( 'NONE', *, *, #39172, .T. ) ;
#25066=CARTESIAN_POINT ( 'NONE',  ( -190.7583438952258916, 294.6698570112193920, -274.9999999999999432 ) ) ;
#25067=CARTESIAN_POINT ( 'NONE',  ( 175.6195620086261613, 290.0000000000001137, -244.9999999999999716 ) ) ;
#25079=CARTESIAN_POINT ( 'NONE',  ( -829.9999999999992042, 430.0000000000002842, -319.9999999999996021 ) ) ;
#25084=DIRECTION ( 'NONE',  ( -0.000000000000000000, -6.938893903907222461E-16, 1.000000000000000000 ) ) ;
#25090=DIRECTION ( 'NONE',  ( 1.000000000000000000, 0.000000000000000000, 0.000000000000000000 ) ) ;
#25098=ORIENTED_EDGE ( 'NONE', *, *, #35167, .F. ) ;
#25121=CARTESIAN_POINT ( 'NONE',  ( -789.9999999999992042, 240.0000000000000853, -360.0000000000000000 ) ) ;
#25125=DIRECTION ( 'NONE',  ( -1.000000000000000000, 0.000000000000000000, 0.000000000000000000 ) ) ;
#25151=EDGE_CURVE ( 'NONE', #26480, #21150, #9901, .T. ) ;
#25171=ORIENTED_EDGE ( 'NONE', *, *, #689, .F. ) ;
#25173=LINE ( 'NONE', #14809, #9326 ) ;
#25197=EDGE_CURVE ( 'NONE', #29001, #14103, #13377, .T. ) ;
#25215=CARTESIAN_POINT ( 'NONE',  ( -200.7583438952258916, 294.6698570112193920, -244.9999999999999716 ) ) ;
#25236=VERTEX_POINT ( 'NONE', #20742 ) ;
#25251=PLANE ( 'NONE',  #40859 ) ;
#25283=ORIENTED_EDGE ( 'NONE', *, *, #4027, .F. ) ;
#25297=VECTOR ( 'NONE', #9581, 1000.000000000000000 ) ;
#25325=DIRECTION ( 'NONE',  ( -1.000000000000000000, -0.000000000000000000, -0.000000000000000000 ) ) ;
#25361=CARTESIAN_POINT ( 'NONE',  ( 879.9999999999992042, 529.9999999999997726, -360.0000000000000000 ) ) ;
#25377=AXIS2_PLACEMENT_3D ( 'NONE', #34731, #3570, #3330 ) ;
#25409=DIRECTION ( 'NONE',  ( -1.000000000000000000, -0.000000000000000000, 0.000000000000000000 ) ) ;
#25412=AXIS2_PLACEMENT_3D ( 'NONE', #37069, #29479, #36398 ) ;
#25465=VECTOR ( 'NONE', #35756, 1000.000000000000000 ) ;
#25480=VECTOR ( 'NONE', #44013, 1000.000000000000000 ) ;
#25492=DIRECTION ( 'NONE',  ( -0.000000000000000000, 0.000000000000000000, -1.000000000000000000 ) ) ;
#25526=EDGE_CURVE ( 'NONE', #25236, #19734, #17491, .T. ) ;
#25547=EDGE_CURVE ( 'NONE', #42263, #19442, #39926, .T. ) ;
#25578=AXIS2_PLACEMENT_3D ( 'NONE', #41104, #6452, #37161 ) ;
#25594=EDGE_CURVE ( 'NONE', #16782, #25236, #43591, .T. ) ;
#25645=ORIENTED_EDGE ( 'NONE', *, *, #9984, .F. ) ;
#25704=FACE_OUTER_BOUND ( 'NONE', #9822, .T. ) ;
#25711=AXIS2_PLACEMENT_3D ( 'NONE', #21183, #32492, #1065 ) ;
#25720=CARTESIAN_POINT ( 'NONE',  ( 265.7583438952258916, 430.0000000000002842, -320.0000000000000000 ) ) ;
#25727=ORIENTED_EDGE ( 'NONE', *, *, #4581, .F. ) ;
#25757=DIRECTION ( 'NONE',  ( 0.000000000000000000, -6.938893903907241197E-16, 1.000000000000000000 ) ) ;
#25768=DIRECTION ( 'NONE',  ( 0.000000000000000000, 0.000000000000000000, -1.000000000000000000 ) ) ;
#25774=CIRCLE ( 'NONE', #19122, 10.00000000000000888 ) ;
#25786=ORIENTED_EDGE ( 'NONE', *, *, #4581, .T. ) ;
#25792=ORIENTED_EDGE ( 'NONE', *, *, #19317, .T. ) ;
#25835=DIRECTION ( 'NONE',  ( 0.000000000000000000, 0.000000000000000000, -1.000000000000000000 ) ) ;
#25845=ORIENTED_EDGE ( 'NONE', *, *, #4114, .F. ) ;
#25881=ADVANCED_FACE ( 'NONE', ( #41275 ), #5926, .F. ) ;
#25882=DIRECTION ( 'NONE',  ( -1.000000000000000000, -0.000000000000000000, -0.000000000000000000 ) ) ;
#25902=ORIENTED_EDGE ( 'NONE', *, *, #40995, .T. ) ;
#25973=CARTESIAN_POINT ( 'NONE',  ( 199.6009925648704098, 290.0000000000001137, -244.9999999999999716 ) ) ;
#25982=CARTESIAN_POINT ( 'NONE',  ( 769.9999999999992042, 240.0000000000000853, -360.0000000000000000 ) ) ;
#26024=CARTESIAN_POINT ( 'NONE',  ( 829.9999999999992042, 290.0000000000001137, -244.9999999999999716 ) ) ;
#26039=EDGE_CURVE ( 'NONE', #39585, #17206, #8941, .T. ) ;
#26065=VERTEX_POINT ( 'NONE', #23011 ) ;
#26077=ORIENTED_EDGE ( 'NONE', *, *, #7473, .F. ) ;
#26142=EDGE_CURVE ( 'NONE', #32851, #42899, #43805, .T. ) ;
#26154=CIRCLE ( 'NONE', #10049, 10.00000000000006395 ) ;
#26170=DIRECTION ( 'NONE',  ( 1.000000000000000000, 0.000000000000000000, 0.000000000000000000 ) ) ;
#26214=PLANE ( 'NONE',  #37988 ) ;
#26225=VECTOR ( 'NONE', #22063, 1000.000000000000000 ) ;
#26253=ORIENTED_EDGE ( 'NONE', *, *, #6286, .T. ) ;
#26255=AXIS2_PLACEMENT_3D ( 'NONE', #9337, #5634, #33149 ) ;
#26272=CARTESIAN_POINT ( 'NONE',  ( 115.7583438952258774, -600.0000000000000000, -320.0000000000000568 ) ) ;
#26273=LINE ( 'NONE', #29068, #17157 ) ;
#26295=FACE_BOUND ( 'NONE', #16988, .T. ) ;
#26301=VECTOR ( 'NONE', #15872, 1000.000000000000000 ) ;
#26366=ADVANCED_FACE ( 'NONE', ( #41499 ), #38271, .F. ) ;
#26471=CARTESIAN_POINT ( 'NONE',  ( 181.9156952255813735, 290.0000000000001137, -244.9999999999999716 ) ) ;
#26480=VERTEX_POINT ( 'NONE', #24381 ) ;
#26505=CARTESIAN_POINT ( 'NONE',  ( -769.9999999999992042, 205.0000000000000568, -339.9999999999999432 ) ) ;
#26514=EDGE_LOOP ( 'NONE', ( #33803, #12294, #16027, #45461 ) ) ;
#26522=VERTEX_POINT ( 'NONE', #13793 ) ;
#26553=DIRECTION ( 'NONE',  ( -1.000000000000000000, -0.000000000000000000, -0.000000000000000000 ) ) ;
#26588=ORIENTED_EDGE ( 'NONE', *, *, #30911, .F. ) ;
#26666=DIRECTION ( 'NONE',  ( -1.000000000000000000, -0.000000000000000000, -0.000000000000000000 ) ) ;
#26667=DIRECTION ( 'NONE',  ( 0.000000000000000000, 0.000000000000000000, -1.000000000000000000 ) ) ;
#26712=EDGE_CURVE ( 'NONE', #22938, #2122, #42646, .T. ) ;
#26740=ORIENTED_EDGE ( 'NONE', *, *, #38540, .F. ) ;
#26746=ORIENTED_EDGE ( 'NONE', *, *, #37612, .F. ) ;
#26816=CARTESIAN_POINT ( 'NONE',  ( -265.7583438952258916, -600.0000000000000000, -320.0000000000000000 ) ) ;
#26834=CARTESIAN_POINT ( 'NONE',  ( -190.7583438952259485, 394.6698570112193920, -274.9999999999999432 ) ) ;
#26858=AXIS2_PLACEMENT_3D ( 'NONE', #23153, #34241, #6075 ) ;
#26872=DIRECTION ( 'NONE',  ( 0.000000000000000000, 1.000000000000000000, -0.000000000000000000 ) ) ;
#26874=ORIENTED_EDGE ( 'NONE', *, *, #17684, .F. ) ;
#26901=AXIS2_PLACEMENT_3D ( 'NONE', #1403, #2077, #36958 ) ;
#26924=VECTOR ( 'NONE', #14928, 1000.000000000000000 ) ;
#26944=DIRECTION ( 'NONE',  ( -1.000000000000000000, 0.000000000000000000, 0.000000000000000000 ) ) ;
#26950=VECTOR ( 'NONE', #34569, 1000.000000000000000 ) ;
#26992=EDGE_CURVE ( 'NONE', #15857, #33458, #44440, .T. ) ;
#27076=CARTESIAN_POINT ( 'NONE',  ( 200.7583438952258916, 294.6698570112193920, -244.9999999999999716 ) ) ;
#27083=CARTESIAN_POINT ( 'NONE',  ( 794.9999999999993179, 240.0000000000000568, -244.9999999999999716 ) ) ;
#27114=ORIENTED_EDGE ( 'NONE', *, *, #7247, .T. ) ;
#27120=DIRECTION ( 'NONE',  ( -1.000000000000000000, -0.000000000000000000, -0.000000000000000000 ) ) ;
#27121=DIRECTION ( 'NONE',  ( -1.000000000000000000, 0.000000000000000000, 0.000000000000000000 ) ) ;
#27130=CARTESIAN_POINT ( 'NONE',  ( 115.7583438952258774, 430.0000000000002842, -320.0000000000000568 ) ) ;
#27153=DIRECTION ( 'NONE',  ( 0.000000000000000000, -1.000000000000000000, -0.000000000000000000 ) ) ;
#27157=VERTEX_POINT ( 'NONE', #2178 ) ;
#27162=DIRECTION ( 'NONE',  ( -0.000000000000000000, 0.000000000000000000, 1.000000000000000000 ) ) ;
#27196=ADVANCED_FACE ( 'NONE', ( #15811 ), #5644, .T. ) ;
#27240=VERTEX_POINT ( 'NONE', #9107 ) ;
#27248=CYLINDRICAL_SURFACE ( 'NONE', #7789, 10.00000000000000888 ) ;
#27260=DIRECTION ( 'NONE',  ( 0.000000000000000000, 0.000000000000000000, 1.000000000000000000 ) ) ;
#27291=DIRECTION ( 'NONE',  ( -0.000000000000000000, 1.000000000000000000, -0.000000000000000000 ) ) ;
#27312=DIRECTION ( 'NONE',  ( 0.000000000000000000, 0.000000000000000000, 1.000000000000000000 ) ) ;
#27370=DIRECTION ( 'NONE',  ( 0.000000000000000000, -0.000000000000000000, 1.000000000000000000 ) ) ;
#27406=CARTESIAN_POINT ( 'NONE',  ( 769.9999999999992042, 205.0000000000000568, -339.9999999999999432 ) ) ;
#27413=CARTESIAN_POINT ( 'NONE',  ( -769.9999999999992042, 205.0000000000000568, -339.9999999999999432 ) ) ;
#27450=DIRECTION ( 'NONE',  ( 1.000000000000000000, -0.000000000000000000, -0.000000000000000000 ) ) ;
#27519=EDGE_CURVE ( 'NONE', #18941, #35125, #28302, .T. ) ;
#27548=ADVANCED_FACE ( 'NONE', ( #17425, #6333 ), #21110, .T. ) ;
#27561=LINE ( 'NONE', #7012, #9554 ) ;
#27579=DIRECTION ( 'NONE',  ( 0.000000000000000000, 0.000000000000000000, 1.000000000000000000 ) ) ;
#27668=VERTEX_POINT ( 'NONE', #27130 ) ;
#27723=EDGE_CURVE ( 'NONE', #12447, #33185, #7952, .T. ) ;
#27741=CARTESIAN_POINT ( 'NONE',  ( 175.6195620086261613, 290.0000000000001137, -244.9999999999999716 ) ) ;
#27783=DIRECTION ( 'NONE',  ( -1.000000000000000000, 0.000000000000000000, 0.000000000000000000 ) ) ;
#27815=CIRCLE ( 'NONE', #3487, 10.00000000000000888 ) ;
#27823=AXIS2_PLACEMENT_3D ( 'NONE', #19474, #16026, #6071 ) ;
#27831=EDGE_CURVE ( 'NONE', #22606, #39117, #3254, .T. ) ;
#27835=CARTESIAN_POINT ( 'NONE',  ( -789.9999999999992042, 205.0000000000000568, -339.9999999999999432 ) ) ;
#27844=CARTESIAN_POINT ( 'NONE',  ( 794.9999999999993179, 205.0000000000000568, -235.0000000000000000 ) ) ;
#27881=EDGE_CURVE ( 'NONE', #7575, #7469, #553, .T. ) ;
#27954=ORIENTED_EDGE ( 'NONE', *, *, #25526, .T. ) ;
#27984=CARTESIAN_POINT ( 'NONE',  ( 794.9999999999993179, 240.0000000000000284, -275.0000000000000000 ) ) ;
#28012=ORIENTED_EDGE ( 'NONE', *, *, #42223, .F. ) ;
#28019=DIRECTION ( 'NONE',  ( 1.000000000000000000, 0.000000000000000000, 0.000000000000000000 ) ) ;
#28139=DIRECTION ( 'NONE',  ( -0.000000000000000000, -0.000000000000000000, 1.000000000000000000 ) ) ;
#28146=PRODUCT_DEFINITION ( 'UNKNOWN', '', #31201, #34424 ) ;
#28149=AXIS2_PLACEMENT_3D ( 'NONE', #21280, #39776, #28898 ) ;
#28161=CARTESIAN_POINT ( 'NONE',  ( 879.9999999999992042, 240.0000000000000853, -360.0000000000000000 ) ) ;
#28175=AXIS2_PLACEMENT_3D ( 'NONE', #12802, #16504, #6100 ) ;
#28202=CARTESIAN_POINT ( 'NONE',  ( 829.9999999999992042, 430.0000000000002842, -320.0000000000000568 ) ) ;
#28204=DIRECTION ( 'NONE',  ( 0.000000000000000000, -6.938893903907241197E-16, 1.000000000000000000 ) ) ;
#28224=CIRCLE ( 'NONE', #1673, 10.00000000000000888 ) ;
#28230=ORIENTED_EDGE ( 'NONE', *, *, #26142, .T. ) ;
#28244=EDGE_LOOP ( 'NONE', ( #17353, #18198, #22256, #33242 ) ) ;
#28249=DIRECTION ( 'NONE',  ( 1.000000000000000000, 0.000000000000000000, 0.000000000000000000 ) ) ;
#28252=DIRECTION ( 'NONE',  ( -0.000000000000000000, 1.000000000000000000, -0.000000000000000000 ) ) ;
#28278=EDGE_CURVE ( 'NONE', #3171, #19734, #43933, .T. ) ;
#28287=VECTOR ( 'NONE', #29915, 1000.000000000000000 ) ;
#28302=CIRCLE ( 'NONE', #25377, 10.00000000000000888 ) ;
#28361=CARTESIAN_POINT ( 'NONE',  ( -829.9999999999992042, 529.9999999999997726, -320.0000000000000000 ) ) ;
#28393=VECTOR ( 'NONE', #15507, 1000.000000000000000 ) ;
#28397=VECTOR ( 'NONE', #37229, 1000.000000000000000 ) ;
#28423=DIRECTION ( 'NONE',  ( 0.000000000000000000, 0.000000000000000000, -1.000000000000000000 ) ) ;
#28443=FACE_OUTER_BOUND ( 'NONE', #9674, .T. ) ;
#28446=DIRECTION ( 'NONE',  ( 0.000000000000000000, -0.000000000000000000, -1.000000000000000000 ) ) ;
#28467=DIRECTION ( 'NONE',  ( 0.000000000000000000, 0.000000000000000000, -1.000000000000000000 ) ) ;
#28479=ORIENTED_EDGE ( 'NONE', *, *, #4345, .F. ) ;
#28511=AXIS2_PLACEMENT_3D ( 'NONE', #38907, #15490, #4253 ) ;
#28559=DIRECTION ( 'NONE',  ( 0.000000000000000000, 0.000000000000000000, 1.000000000000000000 ) ) ;
#28585=CARTESIAN_POINT ( 'NONE',  ( -115.7583438952258774, -600.0000000000000000, -244.9999999999999716 ) ) ;
#28588=ORIENTED_EDGE ( 'NONE', *, *, #40244, .T. ) ;
#28643=EDGE_LOOP ( 'NONE', ( #45586, #26746, #34229, #19248 ) ) ;
#28725=ORIENTED_EDGE ( 'NONE', *, *, #11140, .F. ) ;
#28750=VECTOR ( 'NONE', #42335, 1000.000000000000000 ) ;
#28780=CARTESIAN_POINT ( 'NONE',  ( 784.9999999999992042, 240.0000000000000284, -275.0000000000000000 ) ) ;
#28829=LINE ( 'NONE', #31606, #3938 ) ;
#28832=DIRECTION ( 'NONE',  ( -0.000000000000000000, 1.000000000000000000, -0.000000000000000000 ) ) ;
#28886=LINE ( 'NONE', #10643, #35935 ) ;
#28898=DIRECTION ( 'NONE',  ( 1.000000000000000000, 0.000000000000000000, 0.000000000000000000 ) ) ;
#28934=EDGE_CURVE ( 'NONE', #5389, #30216, #6188, .T. ) ;
#28981=EDGE_CURVE ( 'NONE', #2255, #8421, #42218, .T. ) ;
#28992=ORIENTED_EDGE ( 'NONE', *, *, #25594, .T. ) ;
#28994=ORIENTED_EDGE ( 'NONE', *, *, #14254, .T. ) ;
#29001=VERTEX_POINT ( 'NONE', #7611 ) ;
#29025=CARTESIAN_POINT ( 'NONE',  ( 115.7583438952258774, 430.0000000000002842, -244.9999999999999716 ) ) ;
#29048=ORIENTED_EDGE ( 'NONE', *, *, #9431, .T. ) ;
#29068=CARTESIAN_POINT ( 'NONE',  ( -200.7583438952259485, 394.6698570112193920, -274.9999999999999432 ) ) ;
#29102=AXIS2_PLACEMENT_3D ( 'NONE', #32138, #22192, #11590 ) ;
#29152=AXIS2_PLACEMENT_3D ( 'NONE', #26505, #42985, #11350 ) ;
#29159=EDGE_LOOP ( 'NONE', ( #17650, #17212, #7013, #28725 ) ) ;
#29189=AXIS2_PLACEMENT_3D ( 'NONE', #13340, #41982, #41750 ) ;
#29201=ORIENTED_EDGE ( 'NONE', *, *, #10884, .F. ) ;
#29203=VECTOR ( 'NONE', #13727, 1000.000000000000000 ) ;
#29207=CARTESIAN_POINT ( 'NONE',  ( 789.9999999999992042, 205.0000000000000568, -350.0000000000000000 ) ) ;
#29235=CARTESIAN_POINT ( 'NONE',  ( -190.7583438952259485, 394.6698570112193920, -244.9999999999999716 ) ) ;
#29305=CARTESIAN_POINT ( 'NONE',  ( 769.9999999999992042, 205.0000000000000568, -319.9999999999999432 ) ) ;
#29306=CARTESIAN_POINT ( 'NONE',  ( -769.9999999999992042, 205.0000000000000568, -339.9999999999999432 ) ) ;
#29307=EDGE_CURVE ( 'NONE', #21916, #35390, #8082, .T. ) ;
#29358=EDGE_LOOP ( 'NONE', ( #38847, #23172, #26740, #20935 ) ) ;
#29417=CARTESIAN_POINT ( 'NONE',  ( -879.9999999999992042, 430.0000000000002842, -320.0000000000000568 ) ) ;
#29425=ORIENTED_EDGE ( 'NONE', *, *, #18559, .F. ) ;
#29455=ADVANCED_FACE ( 'NONE', ( #37593 ), #33899, .F. ) ;
#29479=DIRECTION ( 'NONE',  ( 0.000000000000000000, -0.000000000000000000, -1.000000000000000000 ) ) ;
#29480=DIRECTION ( 'NONE',  ( -1.000000000000000000, -0.000000000000000000, -0.000000000000000000 ) ) ;
#29546=DIRECTION ( 'NONE',  ( 1.000000000000000000, -8.326672684688676025E-16, 0.000000000000000000 ) ) ;
#29559=EDGE_CURVE ( 'NONE', #38375, #44144, #9949, .T. ) ;
#29571=DIRECTION ( 'NONE',  ( 0.000000000000000000, 1.000000000000000000, 0.000000000000000000 ) ) ;
#29574=ORIENTED_EDGE ( 'NONE', *, *, #3258, .F. ) ;
#29638=ORIENTED_EDGE ( 'NONE', *, *, #28934, .T. ) ;
#29652=LINE ( 'NONE', #30553, #30055 ) ;
#29655=ORIENTED_EDGE ( 'NONE', *, *, #37131, .F. ) ;
#29715=ORIENTED_EDGE ( 'NONE', *, *, #8274, .F. ) ;
#29735=DIRECTION ( 'NONE',  ( 0.000000000000000000, -1.000000000000000000, -0.000000000000000000 ) ) ;
#29798=CARTESIAN_POINT ( 'NONE',  ( 879.9999999999992042, 529.9999999999997726, -320.0000000000000000 ) ) ;
#29824=PLANE ( 'NONE',  #6491 ) ;
#29849=VECTOR ( 'NONE', #28252, 1000.000000000000000 ) ;
#29878=DIRECTION ( 'NONE',  ( -0.000000000000000000, -0.000000000000000000, 1.000000000000000000 ) ) ;
#29879=ORIENTED_EDGE ( 'NONE', *, *, #44934, .T. ) ;
#29915=DIRECTION ( 'NONE',  ( 0.000000000000000000, -0.000000000000000000, 1.000000000000000000 ) ) ;
#29945=AXIS2_PLACEMENT_3D ( 'NONE', #10240, #27120, #38423 ) ;
#29968=ORIENTED_EDGE ( 'NONE', *, *, #38186, .F. ) ;
#29971=DIRECTION ( 'NONE',  ( 1.000000000000000000, 0.000000000000000000, 0.000000000000000000 ) ) ;
#30014=EDGE_CURVE ( 'NONE', #6928, #42899, #30900, .T. ) ;
#30039=EDGE_CURVE ( 'NONE', #23168, #9031, #847, .T. ) ;
#30055=VECTOR ( 'NONE', #19941, 1000.000000000000000 ) ;
#30071=EDGE_CURVE ( 'NONE', #41324, #18090, #39440, .T. ) ;
#30072=DIRECTION ( 'NONE',  ( 0.000000000000000000, -6.938893903907222461E-16, 1.000000000000000000 ) ) ;
#30104=UNCERTAINTY_MEASURE_WITH_UNIT (LENGTH_MEASURE( 1.000000000000000082E-05 ), #24309, 'distance_accuracy_value', 'NONE');
#30110=ORIENTED_EDGE ( 'NONE', *, *, #45522, .F. ) ;
#30114=ORIENTED_EDGE ( 'NONE', *, *, #30071, .F. ) ;
#30183=CIRCLE ( 'NONE', #5826, 10.00000000000000888 ) ;
#30190=LINE ( 'NONE', #13558, #1647 ) ;
#30215=ORIENTED_EDGE ( 'NONE', *, *, #17684, .T. ) ;
#30216=VERTEX_POINT ( 'NONE', #17956 ) ;
#30221=EDGE_LOOP ( 'NONE', ( #37587, #24412, #17331, #21600 ) ) ;
#30238=EDGE_LOOP ( 'NONE', ( #43632, #20183 ) ) ;
#30318=EDGE_CURVE ( 'NONE', #36817, #32851, #22094, .T. ) ;
#30361=ADVANCED_FACE ( 'NONE', ( #5214 ), #5428, .F. ) ;
#30370=DIRECTION ( 'NONE',  ( 0.000000000000000000, 0.000000000000000000, -1.000000000000000000 ) ) ;
#30395=ORIENTED_EDGE ( 'NONE', *, *, #45233, .F. ) ;
#30408=LINE ( 'NONE', #5463, #21888 ) ;
#30449=ORIENTED_EDGE ( 'NONE', *, *, #20695, .T. ) ;
#30524=EDGE_CURVE ( 'NONE', #1637, #21532, #19094, .T. ) ;
#30527=VECTOR ( 'NONE', #21120, 1000.000000000000000 ) ;
#30553=CARTESIAN_POINT ( 'NONE',  ( 199.6009925648704098, 290.0000000000001137, -274.9999999999999432 ) ) ;
#30611=EDGE_CURVE ( 'NONE', #45491, #18941, #44245, .T. ) ;
#30661=VECTOR ( 'NONE', #32118, 1000.000000000000000 ) ;
#30686=ORIENTED_EDGE ( 'NONE', *, *, #8131, .T. ) ;
#30727=LINE ( 'NONE', #34163, #33136 ) ;
#30761=LINE ( 'NONE', #2569, #5660 ) ;
#30799=EDGE_LOOP ( 'NONE', ( #36926, #41712, #33795, #25063 ) ) ;
#30809=LINE ( 'NONE', #44903, #30661 ) ;
#30818=AXIS2_PLACEMENT_3D ( 'NONE', #13877, #37896, #10175 ) ;
#30841=DIRECTION ( 'NONE',  ( 0.000000000000000000, 0.000000000000000000, 1.000000000000000000 ) ) ;
#30842=LINE ( 'NONE', #35216, #38750 ) ;
#30900=LINE ( 'NONE', #13350, #36487 ) ;
#30911=EDGE_CURVE ( 'NONE', #40516, #16782, #30842, .T. ) ;
#30913=DIRECTION ( 'NONE',  ( -0.000000000000000000, -1.000000000000000000, -0.000000000000000000 ) ) ;
#30915=EDGE_LOOP ( 'NONE', ( #43915, #29048, #25786, #22950 ) ) ;
#30927=ORIENTED_EDGE ( 'NONE', *, *, #9182, .T. ) ;
#30995=CARTESIAN_POINT ( 'NONE',  ( -180.7583438952258348, 394.6698570112193920, -244.9999999999999716 ) ) ;
#31019=DIRECTION ( 'NONE',  ( -1.000000000000000000, -0.000000000000000000, 0.000000000000000000 ) ) ;
#31061=CARTESIAN_POINT ( 'NONE',  ( 829.9999999999992042, 290.0000000000001137, -244.9999999999999716 ) ) ;
#31086=CARTESIAN_POINT ( 'NONE',  ( 829.9999999999992042, -600.0000000000000000, -320.0000000000000568 ) ) ;
#31101=LINE ( 'NONE', #14245, #13536 ) ;
#31201=PRODUCT_DEFINITION_FORMATION_WITH_SPECIFIED_SOURCE ( 'ANY', '', #21103, .NOT_KNOWN. ) ;
#31293=VERTEX_POINT ( 'NONE', #32212 ) ;
#31398=DIRECTION ( 'NONE',  ( -0.000000000000000000, -4.857225732735055920E-15, 1.000000000000000000 ) ) ;
#31440=CARTESIAN_POINT ( 'NONE',  ( -199.6009925648704098, 290.0000000000001137, -244.9999999999999716 ) ) ;
#31469=CARTESIAN_POINT ( 'NONE',  ( -180.7583438952258348, 394.6698570112193920, -274.9999999999999432 ) ) ;
#31484=AXIS2_PLACEMENT_3D ( 'NONE', #28361, #39237, #32998 ) ;
#31503=DIRECTION ( 'NONE',  ( 1.000000000000000000, 0.000000000000000000, -0.000000000000000000 ) ) ;
#31512=CARTESIAN_POINT ( 'NONE',  ( 190.7583438952259485, 394.6698570112193920, -244.9999999999999716 ) ) ;
#31529=FACE_OUTER_BOUND ( 'NONE', #2752, .T. ) ;
#31555=DIRECTION ( 'NONE',  ( -0.000000000000000000, -3.700743415417198493E-16, 1.000000000000000000 ) ) ;
#31606=CARTESIAN_POINT ( 'NONE',  ( 265.7583438952258916, -600.0000000000000000, -320.0000000000000000 ) ) ;
#31686=LINE ( 'NONE', #18694, #32179 ) ;
#31710=LINE ( 'NONE', #32640, #28750 ) ;
#31711=ORIENTED_EDGE ( 'NONE', *, *, #11972, .F. ) ;
#31714=DIRECTION ( 'NONE',  ( 1.000000000000000000, 0.000000000000000000, 0.000000000000000000 ) ) ;
#31780=DIRECTION ( 'NONE',  ( 8.326672684688676025E-16, -1.000000000000000000, 0.000000000000000000 ) ) ;
#31847=CARTESIAN_POINT ( 'NONE',  ( 794.9999999999993179, 205.0000000000000568, -235.0000000000000284 ) ) ;
#31935=ORIENTED_EDGE ( 'NONE', *, *, #39941, .T. ) ;
#32015=ADVANCED_FACE ( 'NONE', ( #20825 ), #17385, .F. ) ;
#32066=ORIENTED_EDGE ( 'NONE', *, *, #38002, .T. ) ;
#32104=ORIENTED_EDGE ( 'NONE', *, *, #7473, .T. ) ;
#32118=DIRECTION ( 'NONE',  ( 0.000000000000000000, 0.000000000000000000, -1.000000000000000000 ) ) ;
#32132=LINE ( 'NONE', #10898, #6744 ) ;
#32138=CARTESIAN_POINT ( 'NONE',  ( 355.8971257818259915, 290.0000000000001137, -244.9999999999999716 ) ) ;
#32141=FACE_OUTER_BOUND ( 'NONE', #41660, .T. ) ;
#32155=VERTEX_POINT ( 'NONE', #36698 ) ;
#32166=EDGE_LOOP ( 'NONE', ( #18595, #39455, #4546, #24949 ) ) ;
#32179=VECTOR ( 'NONE', #21071, 1000.000000000000000 ) ;
#32182=DIRECTION ( 'NONE',  ( 0.000000000000000000, 4.857225732735055920E-15, -1.000000000000000000 ) ) ;
#32198=FACE_OUTER_BOUND ( 'NONE', #19166, .T. ) ;
#32205=CARTESIAN_POINT ( 'NONE',  ( 200.7583438952259485, 394.6698570112193920, -244.9999999999999716 ) ) ;
#32212=CARTESIAN_POINT ( 'NONE',  ( 789.9999999999992042, 240.0000000000000853, -360.0000000000000000 ) ) ;
#32237=VECTOR ( 'NONE', #15650, 1000.000000000000000 ) ;
#32239=DIRECTION ( 'NONE',  ( 1.000000000000000000, 0.000000000000000000, 0.000000000000000000 ) ) ;
#32254=AXIS2_PLACEMENT_3D ( 'NONE', #16047, #40080, #2399 ) ;
#32318=EDGE_CURVE ( 'NONE', #5395, #7469, #31686, .T. ) ;
#32344=DIRECTION ( 'NONE',  ( -1.000000000000000000, -0.000000000000000000, -0.000000000000000000 ) ) ;
#32368=ADVANCED_FACE ( 'NONE', ( #20042, #26295 ), #15899, .T. ) ;
#32408=ORIENTED_EDGE ( 'NONE', *, *, #14716, .F. ) ;
#32436=CARTESIAN_POINT ( 'NONE',  ( -190.7583438952259485, 394.6698570112193920, -274.9999999999999432 ) ) ;
#32456=ORIENTED_EDGE ( 'NONE', *, *, #38309, .T. ) ;
#32492=DIRECTION ( 'NONE',  ( 1.000000000000000000, 0.000000000000000000, -0.000000000000000000 ) ) ;
#32513=ORIENTED_EDGE ( 'NONE', *, *, #9984, .T. ) ;
#32526=LINE ( 'NONE', #25121, #25465 ) ;
#32576=VERTEX_POINT ( 'NONE', #20271 ) ;
#32622=ORIENTED_EDGE ( 'NONE', *, *, #35975, .F. ) ;
#32640=CARTESIAN_POINT ( 'NONE',  ( 115.7583438952258774, 430.0000000000002842, -244.9999999999999716 ) ) ;
#32686=ORIENTED_EDGE ( 'NONE', *, *, #20200, .T. ) ;
#32830=DIRECTION ( 'NONE',  ( 1.000000000000000000, -0.000000000000000000, -0.000000000000000000 ) ) ;
#32850=DIRECTION ( 'NONE',  ( -1.000000000000000000, -0.000000000000000000, 0.000000000000000000 ) ) ;
#32851=VERTEX_POINT ( 'NONE', #38299 ) ;
#32900=CIRCLE ( 'NONE', #43952, 10.00000000000000888 ) ;
#32934=LINE ( 'NONE', #15379, #38811 ) ;
#32940=CARTESIAN_POINT ( 'NONE',  ( 180.7583438952258916, 294.6698570112193920, -244.9999999999999716 ) ) ;
#32976=AXIS2_PLACEMENT_3D ( 'NONE', #42466, #35301, #6894 ) ;
#32998=DIRECTION ( 'NONE',  ( -4.440892098500622217E-15, 1.000000000000000000, 0.000000000000000000 ) ) ;
#32999=FACE_OUTER_BOUND ( 'NONE', #7173, .T. ) ;
#33022=VERTEX_POINT ( 'NONE', #11492 ) ;
#33035=ORIENTED_EDGE ( 'NONE', *, *, #18199, .F. ) ;
#33067=DIRECTION ( 'NONE',  ( 0.000000000000000000, 0.000000000000000000, -1.000000000000000000 ) ) ;
#33100=CARTESIAN_POINT ( 'NONE',  ( 200.7583438952258916, 294.6698570112193920, -274.9999999999999432 ) ) ;
#33114=ADVANCED_FACE ( 'NONE', ( #404 ), #14507, .F. ) ;
#33136=VECTOR ( 'NONE', #23321, 1000.000000000000000 ) ;
#33149=DIRECTION ( 'NONE',  ( 0.000000000000000000, -1.000000000000000000, 1.586032892321651891E-15 ) ) ;
#33185=VERTEX_POINT ( 'NONE', #26471 ) ;
#33204=CARTESIAN_POINT ( 'NONE',  ( -829.9999999999992042, 290.0000000000001705, -319.9999999999996021 ) ) ;
#33230=CARTESIAN_POINT ( 'NONE',  ( 1238.921997096861332, 430.0000000000002842, -320.0000000000000568 ) ) ;
#33242=ORIENTED_EDGE ( 'NONE', *, *, #14716, .T. ) ;
#33274=CARTESIAN_POINT ( 'NONE',  ( 1238.921997096861332, 430.0000000000002842, -320.0000000000000568 ) ) ;
#33291=LINE ( 'NONE', #1636, #9422 ) ;
#33308=DIRECTION ( 'NONE',  ( -0.000000000000000000, 0.000000000000000000, -1.000000000000000000 ) ) ;
#33310=LINE ( 'NONE', #8619, #10657 ) ;
#33313=DIRECTION ( 'NONE',  ( 0.000000000000000000, 1.000000000000000000, 3.700743415417198493E-16 ) ) ;
#33387=DIRECTION ( 'NONE',  ( -1.000000000000000000, -0.000000000000000000, -0.000000000000000000 ) ) ;
#33423=DIRECTION ( 'NONE',  ( 1.000000000000000000, 0.000000000000000000, 0.000000000000000000 ) ) ;
#33454=EDGE_CURVE ( 'NONE', #27157, #36537, #7056, .T. ) ;
#33458=VERTEX_POINT ( 'NONE', #20454 ) ;
#33471=ORIENTED_EDGE ( 'NONE', *, *, #32318, .F. ) ;
#33474=EDGE_CURVE ( 'NONE', #6928, #38375, #34542, .T. ) ;
#33485=AXIS2_PLACEMENT_3D ( 'NONE', #24098, #31503, #45608 ) ;
#33528=ORIENTED_EDGE ( 'NONE', *, *, #17569, .F. ) ;
#33552=DIRECTION ( 'NONE',  ( 0.000000000000000000, 0.000000000000000000, 1.000000000000000000 ) ) ;
#33553=AXIS2_PLACEMENT_3D ( 'NONE', #40044, #33552, #26170 ) ;
#33569=DIRECTION ( 'NONE',  ( -1.000000000000000000, 0.000000000000000000, 0.000000000000000000 ) ) ;
#33606=DIRECTION ( 'NONE',  ( 1.000000000000000000, 0.000000000000000000, 0.000000000000000000 ) ) ;
#33694=VERTEX_POINT ( 'NONE', #35223 ) ;
#33795=ORIENTED_EDGE ( 'NONE', *, *, #18559, .T. ) ;
#33801=ORIENTED_EDGE ( 'NONE', *, *, #34615, .T. ) ;
#33803=ORIENTED_EDGE ( 'NONE', *, *, #34811, .F. ) ;
#33820=DIRECTION ( 'NONE',  ( -0.000000000000000000, -1.000000000000000000, -0.000000000000000000 ) ) ;
#33843=CARTESIAN_POINT ( 'NONE',  ( -789.9999999999992042, 205.0000000000000568, -339.9999999999999432 ) ) ;
#33882=CARTESIAN_POINT ( 'NONE',  ( 769.9999999999992042, 240.0000000000000568, -319.9999999999999432 ) ) ;
#33899=PLANE ( 'NONE',  #41674 ) ;
#33925=ORIENTED_EDGE ( 'NONE', *, *, #23560, .T. ) ;
#33928=CARTESIAN_POINT ( 'NONE',  ( 769.9999999999992042, 240.0000000000000853, -360.0000000000000000 ) ) ;
#34001=CARTESIAN_POINT ( 'NONE',  ( -200.7583438952259485, 394.6698570112193920, -274.9999999999999432 ) ) ;
#34080=ORIENTED_EDGE ( 'NONE', *, *, #33474, .F. ) ;
#34103=DIRECTION ( 'NONE',  ( -0.000000000000000000, -0.000000000000000000, 1.000000000000000000 ) ) ;
#34120=CARTESIAN_POINT ( 'NONE',  ( 784.9999999999992042, 205.0000000000000568, -255.0000000000000000 ) ) ;
#34163=CARTESIAN_POINT ( 'NONE',  ( -879.9999999999992042, 529.9999999999997726, -244.9999999999999716 ) ) ;
#34179=VECTOR ( 'NONE', #1294, 1000.000000000000000 ) ;
#34229=ORIENTED_EDGE ( 'NONE', *, *, #29559, .F. ) ;
#34240=ORIENTED_EDGE ( 'NONE', *, *, #27881, .F. ) ;
#34241=DIRECTION ( 'NONE',  ( 0.000000000000000000, 0.000000000000000000, 1.000000000000000000 ) ) ;
#34244=AXIS2_PLACEMENT_3D ( 'NONE', #26834, #2355, #12327 ) ;
#34259=LINE ( 'NONE', #16492, #7043 ) ;
#34274=EDGE_CURVE ( 'NONE', #8204, #36310, #5618, .T. ) ;
#34285=EDGE_CURVE ( 'NONE', #10220, #45115, #40959, .T. ) ;
#34305=VERTEX_POINT ( 'NONE', #16470 ) ;
#34323=CARTESIAN_POINT ( 'NONE',  ( 879.9999999999992042, 240.0000000000000568, -244.9999999999999716 ) ) ;
#34333=EDGE_CURVE ( 'NONE', #13729, #12447, #29652, .T. ) ;
#34336=CARTESIAN_POINT ( 'NONE',  ( -180.7583438952258916, 294.6698570112193920, -274.9999999999999432 ) ) ;
#34347=AXIS2_PLACEMENT_3D ( 'NONE', #17474, #31555, #45655 ) ;
#34399=DIRECTION ( 'NONE',  ( 0.000000000000000000, 0.000000000000000000, 1.000000000000000000 ) ) ;
#34405=LINE ( 'NONE', #6684, #35791 ) ;
#34424=PRODUCT_DEFINITION_CONTEXT ( 'detailed design', #21377, 'design' ) ;
#34502=ADVANCED_FACE ( 'NONE', ( #37026 ), #5380, .T. ) ;
#34504=VERTEX_POINT ( 'NONE', #24528 ) ;
#34515=CARTESIAN_POINT ( 'NONE',  ( 769.9999999999992042, 205.0000000000000568, -319.9999999999999432 ) ) ;
#34542=LINE ( 'NONE', #27844, #6152 ) ;
#34569=DIRECTION ( 'NONE',  ( -1.000000000000000000, -0.000000000000000000, -0.000000000000000000 ) ) ;
#34578=DIRECTION ( 'NONE',  ( -5.551115123125783688E-16, -1.000000000000000000, 0.000000000000000000 ) ) ;
#34581=ADVANCED_FACE ( 'NONE', ( #20390, #34935 ), #10226, .F. ) ;
#34605=CARTESIAN_POINT ( 'NONE',  ( 794.9999999999993179, 205.0000000000000568, -245.0000000000000284 ) ) ;
#34615=EDGE_CURVE ( 'NONE', #8204, #27240, #41196, .T. ) ;
#34642=CIRCLE ( 'NONE', #44233, 10.00000000000000888 ) ;
#34645=DIRECTION ( 'NONE',  ( 1.000000000000000000, 0.000000000000000000, 0.000000000000000000 ) ) ;
#34728=ORIENTED_EDGE ( 'NONE', *, *, #20468, .T. ) ;
#34731=CARTESIAN_POINT ( 'NONE',  ( -190.7583438952258916, 294.6698570112193920, -244.9999999999999716 ) ) ;
#34789=FACE_OUTER_BOUND ( 'NONE', #42809, .T. ) ;
#34811=EDGE_CURVE ( 'NONE', #13136, #44609, #17159, .T. ) ;
#34852=AXIS2_PLACEMENT_3D ( 'NONE', #17990, #4804, #18672 ) ;
#34892=PLANE ( 'NONE',  #21164 ) ;
#34895=ORIENTED_EDGE ( 'NONE', *, *, #37612, .T. ) ;
#34935=FACE_BOUND ( 'NONE', #30238, .T. ) ;
#35028=CARTESIAN_POINT ( 'NONE',  ( 769.9999999999992042, 205.0000000000000568, -319.9999999999999432 ) ) ;
#35029=CYLINDRICAL_SURFACE ( 'NONE', #19054, 9.999999999999980460 ) ;
#35099=ORIENTED_EDGE ( 'NONE', *, *, #19367, .T. ) ;
#35112=EDGE_CURVE ( 'NONE', #25018, #5395, #11371, .T. ) ;
#35125=VERTEX_POINT ( 'NONE', #25215 ) ;
#35136=DIRECTION ( 'NONE',  ( -0.000000000000000000, -4.857225732735055920E-15, 1.000000000000000000 ) ) ;
#35141=ADVANCED_FACE ( 'NONE', ( #12283, #5563 ), #29824, .F. ) ;
#35167=EDGE_CURVE ( 'NONE', #21532, #66, #36534, .T. ) ;
#35185=DIRECTION ( 'NONE',  ( 0.000000000000000000, 0.000000000000000000, 1.000000000000000000 ) ) ;
#35216=CARTESIAN_POINT ( 'NONE',  ( 1238.921997096861332, 579.9999999999998863, -360.0000000000000000 ) ) ;
#35223=CARTESIAN_POINT ( 'NONE',  ( -265.7583438952257779, 430.0000000000002842, -320.0000000000000568 ) ) ;
#35225=ORIENTED_EDGE ( 'NONE', *, *, #34333, .T. ) ;
#35233=AXIS2_PLACEMENT_3D ( 'NONE', #6246, #24018, #2317 ) ;
#35238=DIRECTION ( 'NONE',  ( -1.000000000000000000, 0.000000000000000000, 0.000000000000000000 ) ) ;
#35247=LINE ( 'NONE', #20693, #26950 ) ;
#35252=PLANE ( 'NONE',  #43007 ) ;
#35301=DIRECTION ( 'NONE',  ( 1.000000000000000000, 0.000000000000000000, 0.000000000000000000 ) ) ;
#35364=LINE ( 'NONE', #37924, #45314 ) ;
#35390=VERTEX_POINT ( 'NONE', #44362 ) ;
#35398=EDGE_CURVE ( 'NONE', #38320, #45077, #33291, .T. ) ;
#35439=ADVANCED_FACE ( 'NONE', ( #41145 ), #17330, .F. ) ;
#35453=EDGE_LOOP ( 'NONE', ( #38636, #21837, #28230, #23663 ) ) ;
#35462=EDGE_LOOP ( 'NONE', ( #29201, #25283, #16247, #39047 ) ) ;
#35479=ADVANCED_FACE ( 'NONE', ( #37664 ), #13199, .T. ) ;
#35514=DIRECTION ( 'NONE',  ( 1.000000000000000000, 0.000000000000000000, 0.000000000000000000 ) ) ;
#35584=CARTESIAN_POINT ( 'NONE',  ( -199.6009925648704098, 290.0000000000001137, -274.9999999999999432 ) ) ;
#35603=ORIENTED_EDGE ( 'NONE', *, *, #13412, .F. ) ;
#35623=EDGE_LOOP ( 'NONE', ( #20622, #10334, #11092, #38764, #45206, #43076 ) ) ;
#35628=DIRECTION ( 'NONE',  ( 0.000000000000000000, -1.000000000000000000, -4.857225732735055920E-15 ) ) ;
#35643=VECTOR ( 'NONE', #41680, 1000.000000000000000 ) ;
#35683=EDGE_CURVE ( 'NONE', #22016, #7575, #45525, .T. ) ;
#35687=CARTESIAN_POINT ( 'NONE',  ( -190.7583438952259485, 394.6698570112193920, -274.9999999999999432 ) ) ;
#35732=ORIENTED_EDGE ( 'NONE', *, *, #34285, .T. ) ;
#35733=VECTOR ( 'NONE', #13586, 1000.000000000000000 ) ;
#35756=DIRECTION ( 'NONE',  ( 0.000000000000000000, 1.000000000000000000, 0.000000000000000000 ) ) ;
#35791=VECTOR ( 'NONE', #5991, 1000.000000000000000 ) ;
#35818=CIRCLE ( 'NONE', #9172, 50.00000000000004263 ) ;
#35864=ORIENTED_EDGE ( 'NONE', *, *, #35975, .T. ) ;
#35868=EDGE_LOOP ( 'NONE', ( #23847, #4857, #30395, #5381 ) ) ;
#35879=ORIENTED_EDGE ( 'NONE', *, *, #25526, .F. ) ;
#35887=LINE ( 'NONE', #29417, #41770 ) ;
#35930=ORIENTED_EDGE ( 'NONE', *, *, #43865, .F. ) ;
#35935=VECTOR ( 'NONE', #28423, 1000.000000000000000 ) ;
#35970=ORIENTED_EDGE ( 'NONE', *, *, #5113, .T. ) ;
#35975=EDGE_CURVE ( 'NONE', #36814, #32576, #24938, .T. ) ;
#35977=ORIENTED_EDGE ( 'NONE', *, *, #12855, .T. ) ;
#36019=ORIENTED_EDGE ( 'NONE', *, *, #30611, .T. ) ;
#36135=ORIENTED_EDGE ( 'NONE', *, *, #4112, .T. ) ;
#36199=ORIENTED_EDGE ( 'NONE', *, *, #27723, .F. ) ;
#36207=DIRECTION ( 'NONE',  ( 1.000000000000000000, -0.000000000000000000, -0.000000000000000000 ) ) ;
#36215=DIRECTION ( 'NONE',  ( -0.000000000000000000, -0.000000000000000000, -1.000000000000000000 ) ) ;
#36220=ORIENTED_EDGE ( 'NONE', *, *, #44416, .F. ) ;
#36240=EDGE_CURVE ( 'NONE', #24825, #25236, #2473, .T. ) ;
#36277=LINE ( 'NONE', #4202, #35643 ) ;
#36285=CARTESIAN_POINT ( 'NONE',  ( 190.7583438952258916, 294.6698570112193920, -274.9999999999999432 ) ) ;
#36297=ADVANCED_FACE ( 'NONE', ( #20932 ), #35029, .F. ) ;
#36310=VERTEX_POINT ( 'NONE', #41752 ) ;
#36324=CARTESIAN_POINT ( 'NONE',  ( 829.9999999999992042, 529.9999999999997726, -360.0000000000000000 ) ) ;
#36337=CARTESIAN_POINT ( 'NONE',  ( -789.9999999999989768, 240.0000000000000853, -360.0000000000000000 ) ) ;
#36398=DIRECTION ( 'NONE',  ( 1.000000000000000000, 0.000000000000000000, 0.000000000000000000 ) ) ;
#36431=LINE ( 'NONE', #2390, #3661 ) ;
#36437=CYLINDRICAL_SURFACE ( 'NONE', #20388, 10.00000000000000888 ) ;
#36440=DIRECTION ( 'NONE',  ( -0.000000000000000000, -0.000000000000000000, 1.000000000000000000 ) ) ;
#36443=ORIENTED_EDGE ( 'NONE', *, *, #30014, .T. ) ;
#36487=VECTOR ( 'NONE', #25325, 1000.000000000000000 ) ;
#36517=AXIS2_PLACEMENT_3D ( 'NONE', #15157, #40329, #43989 ) ;
#36534=LINE ( 'NONE', #22425, #10179 ) ;
#36537=VERTEX_POINT ( 'NONE', #29025 ) ;
#36556=ORIENTED_EDGE ( 'NONE', *, *, #2120, .F. ) ;
#36582=AXIS2_PLACEMENT_3D ( 'NONE', #10944, #76, #17648 ) ;
#36598=AXIS2_PLACEMENT_3D ( 'NONE', #34120, #43832, #16595 ) ;
#36619=VECTOR ( 'NONE', #30072, 1000.000000000000000 ) ;
#36639=DIRECTION ( 'NONE',  ( 0.000000000000000000, 0.000000000000000000, 1.000000000000000000 ) ) ;
#36652=ORIENTED_EDGE ( 'NONE', *, *, #37131, .T. ) ;
#36698=CARTESIAN_POINT ( 'NONE',  ( -265.7583438952258916, 290.0000000000001137, -320.0000000000000568 ) ) ;
#36744=EDGE_CURVE ( 'NONE', #19442, #26065, #42690, .T. ) ;
#36770=ORIENTED_EDGE ( 'NONE', *, *, #24413, .T. ) ;
#36787=CARTESIAN_POINT ( 'NONE',  ( 1238.921997096861332, 240.0000000000000853, -360.0000000000000000 ) ) ;
#36814=VERTEX_POINT ( 'NONE', #45095 ) ;
#36817=VERTEX_POINT ( 'NONE', #27083 ) ;
#36861=DIRECTION ( 'NONE',  ( 0.000000000000000000, -0.000000000000000000, 1.000000000000000000 ) ) ;
#36926=ORIENTED_EDGE ( 'NONE', *, *, #14579, .F. ) ;
#36958=DIRECTION ( 'NONE',  ( -1.000000000000000000, 0.000000000000000000, -0.000000000000000000 ) ) ;
#36997=CARTESIAN_POINT ( 'NONE',  ( -879.9999999999992042, 579.9999999999998863, -320.0000000000000000 ) ) ;
#37026=FACE_OUTER_BOUND ( 'NONE', #30221, .T. ) ;
#37031=ADVANCED_FACE ( 'NONE', ( #22530 ), #23594, .F. ) ;
#37062=CARTESIAN_POINT ( 'NONE',  ( -879.9999999999992042, 240.0000000000002274, -244.9999999999999716 ) ) ;
#37069=CARTESIAN_POINT ( 'NONE',  ( -829.9999999999992042, 529.9999999999997726, -360.0000000000000000 ) ) ;
#37091=ORIENTED_EDGE ( 'NONE', *, *, #6607, .T. ) ;
#37112=VERTEX_POINT ( 'NONE', #27984 ) ;
#37131=EDGE_CURVE ( 'NONE', #35125, #34305, #17372, .T. ) ;
#37145=ORIENTED_EDGE ( 'NONE', *, *, #42510, .T. ) ;
#37161=DIRECTION ( 'NONE',  ( -1.000000000000000000, 0.000000000000000000, -0.000000000000000000 ) ) ;
#37165=VERTEX_POINT ( 'NONE', #14366 ) ;
#37208=ORIENTED_EDGE ( 'NONE', *, *, #43865, .T. ) ;
#37218=CLOSED_SHELL ( 'NONE', ( #36297, #18231, #2134, #9320, #2666, #15122, #30361, #8922, #189, #16424, #37359, #29455, #2898, #1683, #16249, #35439, #25881, #45301, #33114, #14549, #39690, #13990, #26366, #10564, #43923, #42743, #4877, #9473, #32015, #23787, #41864, #1558, #39989, #21946, #2662, #21867, #35479, #34502, #23017, #22066, #35141, #19895, #27548, #6374, #14244, #11532, #11354, #39414, #34581, #32368, #18807, #10276, #9724, #37031, #15944, #27196 ) ) ;
#37229=DIRECTION ( 'NONE',  ( -0.000000000000000000, 1.000000000000000000, -1.586032892321652088E-15 ) ) ;
#37250=VECTOR ( 'NONE', #26666, 1000.000000000000000 ) ;
#37297=CARTESIAN_POINT ( 'NONE',  ( -265.7583438952258916, -600.0000000000000000, -244.9999999999999716 ) ) ;
#37304=DIRECTION ( 'NONE',  ( 1.000000000000000000, 0.000000000000000000, -0.000000000000000000 ) ) ;
#37331=CIRCLE ( 'NONE', #13746, 10.00000000000000888 ) ;
#37350=DIRECTION ( 'NONE',  ( 0.000000000000000000, -6.938893903907222461E-16, 1.000000000000000000 ) ) ;
#37359=ADVANCED_FACE ( 'NONE', ( #32141 ), #21509, .F. ) ;
#37380=AXIS2_PLACEMENT_3D ( 'NONE', #26816, #40921, #33308 ) ;
#37402=CARTESIAN_POINT ( 'NONE',  ( 829.9999999999992042, 579.9999999999998863, -320.0000000000000000 ) ) ;
#37410=VECTOR ( 'NONE', #33569, 1000.000000000000000 ) ;
#37479=FACE_OUTER_BOUND ( 'NONE', #7937, .T. ) ;
#37540=VECTOR ( 'NONE', #44582, 1000.000000000000000 ) ;
#37570=CARTESIAN_POINT ( 'NONE',  ( 879.9999999999992042, 239.9999999999998863, -244.9999999999999716 ) ) ;
#37571=DIRECTION ( 'NONE',  ( 0.000000000000000000, 0.000000000000000000, -1.000000000000000000 ) ) ;
#37587=ORIENTED_EDGE ( 'NONE', *, *, #20468, .F. ) ;
#37593=FACE_OUTER_BOUND ( 'NONE', #18724, .T. ) ;
#37612=EDGE_CURVE ( 'NONE', #44144, #16382, #735, .T. ) ;
#37640=FACE_BOUND ( 'NONE', #1804, .T. ) ;
#37644=EDGE_CURVE ( 'NONE', #23168, #13136, #25774, .T. ) ;
#37664=FACE_OUTER_BOUND ( 'NONE', #35868, .T. ) ;
#37668=EDGE_CURVE ( 'NONE', #26480, #8204, #15439, .T. ) ;
#37675=ORIENTED_EDGE ( 'NONE', *, *, #39050, .F. ) ;
#37684=DIRECTION ( 'NONE',  ( 0.000000000000000000, 0.000000000000000000, -1.000000000000000000 ) ) ;
#37692=( LENGTH_UNIT ( ) NAMED_UNIT ( * ) SI_UNIT ( .MILLI., .METRE. ) );
#37695=CARTESIAN_POINT ( 'NONE',  ( 829.9999999999992042, 430.0000000000002842, -244.9999999999999716 ) ) ;
#37710=DIRECTION ( 'NONE',  ( -1.000000000000000000, 0.000000000000000000, 0.000000000000000000 ) ) ;
#37730=ORIENTED_EDGE ( 'NONE', *, *, #10884, .T. ) ;
#37740=CARTESIAN_POINT ( 'NONE',  ( 265.7583438952258916, 290.0000000000001137, -244.9999999999999716 ) ) ;
#37760=CARTESIAN_POINT ( 'NONE',  ( -181.9156952255813735, 290.0000000000001137, -244.9999999999999716 ) ) ;
#37809=CARTESIAN_POINT ( 'NONE',  ( -115.7583438952258774, -600.0000000000000000, -320.0000000000000568 ) ) ;
#37854=PLANE ( 'NONE',  #25578 ) ;
#37859=ORIENTED_EDGE ( 'NONE', *, *, #11150, .T. ) ;
#37896=DIRECTION ( 'NONE',  ( -0.000000000000000000, 0.000000000000000000, 1.000000000000000000 ) ) ;
#37913=CARTESIAN_POINT ( 'NONE',  ( 879.9999999999992042, 430.0000000000002842, -320.0000000000000568 ) ) ;
#37924=CARTESIAN_POINT ( 'NONE',  ( 879.9999999999992042, 240.0000000000000853, -360.0000000000000000 ) ) ;
#37938=VECTOR ( 'NONE', #25835, 1000.000000000000000 ) ;
#37945=EDGE_CURVE ( 'NONE', #19734, #43685, #30727, .T. ) ;
#37988=AXIS2_PLACEMENT_3D ( 'NONE', #15594, #12132, #43537 ) ;
#38002=EDGE_CURVE ( 'NONE', #1656, #27157, #5312, .T. ) ;
#38008=DIRECTION ( 'NONE',  ( -1.000000000000000000, -0.000000000000000000, 0.000000000000000000 ) ) ;
#38034=CARTESIAN_POINT ( 'NONE',  ( -789.9999999999992042, 205.0000000000000568, -329.9999999999999432 ) ) ;
#38113=CARTESIAN_POINT ( 'NONE',  ( 180.7583438952258348, 394.6698570112193920, -274.9999999999999432 ) ) ;
#38114=EDGE_CURVE ( 'NONE', #26522, #45491, #30183, .T. ) ;
#38140=VECTOR ( 'NONE', #36215, 1000.000000000000000 ) ;
#38150=CARTESIAN_POINT ( 'NONE',  ( -265.7583438952258916, 290.0000000000001137, -244.9999999999999716 ) ) ;
#38186=EDGE_CURVE ( 'NONE', #5395, #18090, #9253, .T. ) ;
#38203=DIRECTION ( 'NONE',  ( -1.000000000000000000, 0.000000000000000000, 0.000000000000000000 ) ) ;
#38211=VECTOR ( 'NONE', #27783, 1000.000000000000000 ) ;
#38240=ORIENTED_EDGE ( 'NONE', *, *, #23484, .T. ) ;
#38271=CYLINDRICAL_SURFACE ( 'NONE', #41817, 10.00000000000006395 ) ;
#38299=CARTESIAN_POINT ( 'NONE',  ( 784.9999999999992042, 239.9999999999999432, -244.9999999999999716 ) ) ;
#38306=ORIENTED_EDGE ( 'NONE', *, *, #30524, .T. ) ;
#38309=EDGE_CURVE ( 'NONE', #22342, #39117, #41572, .T. ) ;
#38320=VERTEX_POINT ( 'NONE', #6689 ) ;
#38375=VERTEX_POINT ( 'NONE', #31847 ) ;
#38387=DIRECTION ( 'NONE',  ( 1.000000000000000000, 0.000000000000000000, 0.000000000000000000 ) ) ;
#38412=ORIENTED_EDGE ( 'NONE', *, *, #27831, .F. ) ;
#38423=DIRECTION ( 'NONE',  ( 0.000000000000000000, 0.000000000000000000, 1.000000000000000000 ) ) ;
#38428=DIRECTION ( 'NONE',  ( 0.000000000000000000, 0.000000000000000000, -1.000000000000000000 ) ) ;
#38439=CARTESIAN_POINT ( 'NONE',  ( -829.9999999999992042, -600.0000000000000000, -319.9999999999996021 ) ) ;
#38457=EDGE_LOOP ( 'NONE', ( #44856, #19366, #45363, #38591 ) ) ;
#38499=CARTESIAN_POINT ( 'NONE',  ( 1238.921997096861332, 579.9999999999998863, -320.0000000000000000 ) ) ;
#38502=VERTEX_POINT ( 'NONE', #28161 ) ;
#38536=EDGE_CURVE ( 'NONE', #3087, #35125, #36431, .T. ) ;
#38540=EDGE_CURVE ( 'NONE', #9031, #44609, #34642, .T. ) ;
#38556=CARTESIAN_POINT ( 'NONE',  ( 794.9999999999993179, 239.9999999999998863, -235.0000000000000000 ) ) ;
#38591=ORIENTED_EDGE ( 'NONE', *, *, #16520, .T. ) ;
#38636=ORIENTED_EDGE ( 'NONE', *, *, #44758, .F. ) ;
#38653=CARTESIAN_POINT ( 'NONE',  ( -769.9999999999992042, 240.0000000000000568, -319.9999999999999432 ) ) ;
#38732=VECTOR ( 'NONE', #31398, 1000.000000000000000 ) ;
#38742=CYLINDRICAL_SURFACE ( 'NONE', #19342, 10.00000000000000888 ) ;
#38746=CIRCLE ( 'NONE', #36517, 10.00000000000000888 ) ;
#38750=VECTOR ( 'NONE', #16527, 1000.000000000000000 ) ;
#38764=ORIENTED_EDGE ( 'NONE', *, *, #15112, .T. ) ;
#38811=VECTOR ( 'NONE', #5873, 1000.000000000000000 ) ;
#38818=EDGE_CURVE ( 'NONE', #27240, #18651, #27561, .T. ) ;
#38823=AXIS2_PLACEMENT_3D ( 'NONE', #18388, #38959, #7309 ) ;
#38847=ORIENTED_EDGE ( 'NONE', *, *, #37644, .T. ) ;
#38867=CARTESIAN_POINT ( 'NONE',  ( -181.9156952255813735, 290.0000000000001137, -274.9999999999999432 ) ) ;
#38886=EDGE_LOOP ( 'NONE', ( #7302, #30449 ) ) ;
#38889=ORIENTED_EDGE ( 'NONE', *, *, #27881, .T. ) ;
#38907=CARTESIAN_POINT ( 'NONE',  ( -829.9999999999992042, -600.0000000000000000, -319.9999999999996021 ) ) ;
#38915=CARTESIAN_POINT ( 'NONE',  ( 784.9999999999992042, 205.0000000000000568, -274.9999999999999432 ) ) ;
#38917=EDGE_CURVE ( 'NONE', #3087, #7747, #25043, .T. ) ;
#38925=AXIS2_PLACEMENT_3D ( 'NONE', #13931, #31019, #44654 ) ;
#38959=DIRECTION ( 'NONE',  ( 1.000000000000000000, 0.000000000000000000, 0.000000000000000000 ) ) ;
#38960=CYLINDRICAL_SURFACE ( 'NONE', #1137, 10.00000000000006395 ) ;
#39011=LINE ( 'NONE', #20965, #42276 ) ;
#39017=CARTESIAN_POINT ( 'NONE',  ( -180.7583438952258916, 294.6698570112193920, -274.9999999999999432 ) ) ;
#39047=ORIENTED_EDGE ( 'NONE', *, *, #22135, .F. ) ;
#39050=EDGE_CURVE ( 'NONE', #6536, #37165, #17173, .T. ) ;
#39080=DIRECTION ( 'NONE',  ( -1.000000000000000000, -0.000000000000000000, -0.000000000000000000 ) ) ;
#39117=VERTEX_POINT ( 'NONE', #13722 ) ;
#39134=DIRECTION ( 'NONE',  ( 1.000000000000000000, 0.000000000000000000, 0.000000000000000000 ) ) ;
#39153=LINE ( 'NONE', #10974, #42432 ) ;
#39172=EDGE_CURVE ( 'NONE', #36537, #27668, #31710, .T. ) ;
#39180=DIRECTION ( 'NONE',  ( 1.000000000000000000, 0.000000000000000000, 0.000000000000000000 ) ) ;
#39237=DIRECTION ( 'NONE',  ( -0.000000000000000000, -3.700743415417198493E-16, 1.000000000000000000 ) ) ;
#39284=DIRECTION ( 'NONE',  ( -1.000000000000000000, -0.000000000000000000, -0.000000000000000000 ) ) ;
#39361=DIRECTION ( 'NONE',  ( -8.326672684688676025E-16, -1.000000000000000000, 0.000000000000000000 ) ) ;
#39414=ADVANCED_FACE ( 'NONE', ( #983 ), #18101, .F. ) ;
#39432=CARTESIAN_POINT ( 'NONE',  ( 769.9999999999992042, 205.0000000000000568, -339.9999999999999432 ) ) ;
#39440=LINE ( 'NONE', #18871, #18071 ) ;
#39455=ORIENTED_EDGE ( 'NONE', *, *, #114, .F. ) ;
#39541=VECTOR ( 'NONE', #7998, 1000.000000000000000 ) ;
#39585=VERTEX_POINT ( 'NONE', #33100 ) ;
#39604=DIRECTION ( 'NONE',  ( 0.000000000000000000, -1.000000000000000000, 0.000000000000000000 ) ) ;
#39611=CARTESIAN_POINT ( 'NONE',  ( -879.9999999999992042, 240.0000000000000853, -360.0000000000000000 ) ) ;
#39644=FACE_OUTER_BOUND ( 'NONE', #32166, .T. ) ;
#39656=CARTESIAN_POINT ( 'NONE',  ( 115.7583438952258774, -600.0000000000000000, -244.9999999999999716 ) ) ;
#39690=ADVANCED_FACE ( 'NONE', ( #15323 ), #12736, .F. ) ;
#39715=CARTESIAN_POINT ( 'NONE',  ( -265.7583438952258916, 430.0000000000002842, -320.0000000000000000 ) ) ;
#39776=DIRECTION ( 'NONE',  ( 0.000000000000000000, 0.000000000000000000, 1.000000000000000000 ) ) ;
#39924=LINE ( 'NONE', #8057, #43918 ) ;
#39926=LINE ( 'NONE', #29305, #10094 ) ;
#39927=CYLINDRICAL_SURFACE ( 'NONE', #15274, 20.00000000000001776 ) ;
#39941=EDGE_CURVE ( 'NONE', #37112, #12764, #30761, .T. ) ;
#39971=VERTEX_POINT ( 'NONE', #38150 ) ;
#39989=ADVANCED_FACE ( 'NONE', ( #24031 ), #34892, .F. ) ;
#40044=CARTESIAN_POINT ( 'NONE',  ( 190.7583438952258916, 294.6698570112193920, -274.9999999999999432 ) ) ;
#40080=DIRECTION ( 'NONE',  ( 0.000000000000000000, 0.000000000000000000, -1.000000000000000000 ) ) ;
#40140=LINE ( 'NONE', #39715, #38140 ) ;
#40164=AXIS2_PLACEMENT_3D ( 'NONE', #1725, #37304, #36639 ) ;
#40198=CIRCLE ( 'NONE', #33553, 10.00000000000000888 ) ;
#40216=PLANE ( 'NONE',  #26901 ) ;
#40244=EDGE_CURVE ( 'NONE', #4463, #29001, #28886, .T. ) ;
#40255=ORIENTED_EDGE ( 'NONE', *, *, #17246, .T. ) ;
#40266=ORIENTED_EDGE ( 'NONE', *, *, #23550, .T. ) ;
#40329=DIRECTION ( 'NONE',  ( 1.000000000000000000, 0.000000000000000000, 0.000000000000000000 ) ) ;
#40338=DIRECTION ( 'NONE',  ( -0.000000000000000000, 1.000000000000000000, -0.000000000000000000 ) ) ;
#40432=ORIENTED_EDGE ( 'NONE', *, *, #42547, .F. ) ;
#40516=VERTEX_POINT ( 'NONE', #24954 ) ;
#40541=FACE_OUTER_BOUND ( 'NONE', #12164, .T. ) ;
#40548=LINE ( 'NONE', #16282, #22414 ) ;
#40622=EDGE_LOOP ( 'NONE', ( #35879, #40863, #16995, #10572 ) ) ;
#40627=ORIENTED_EDGE ( 'NONE', *, *, #29559, .T. ) ;
#40657=LINE ( 'NONE', #33274, #28393 ) ;
#40703=VECTOR ( 'NONE', #5143, 1000.000000000000000 ) ;
#40704=LINE ( 'NONE', #15767, #28397 ) ;
#40775=PLANE ( 'NONE',  #1822 ) ;
#40780=ORIENTED_EDGE ( 'NONE', *, *, #44081, .T. ) ;
#40787=ORIENTED_EDGE ( 'NONE', *, *, #22360, .T. ) ;
#40798=EDGE_CURVE ( 'NONE', #6536, #6383, #22173, .T. ) ;
#40859=AXIS2_PLACEMENT_3D ( 'NONE', #784, #39604, #43711 ) ;
#40863=ORIENTED_EDGE ( 'NONE', *, *, #25594, .F. ) ;
#40901=CARTESIAN_POINT ( 'NONE',  ( 789.9999999999992042, 205.0000000000000568, -339.9999999999999432 ) ) ;
#40921=DIRECTION ( 'NONE',  ( 1.000000000000000000, 0.000000000000000000, -0.000000000000000000 ) ) ;
#40941=VECTOR ( 'NONE', #27153, 1000.000000000000000 ) ;
#40959=LINE ( 'NONE', #1470, #37410 ) ;
#40995=EDGE_CURVE ( 'NONE', #15857, #3171, #12682, .T. ) ;
#41104=CARTESIAN_POINT ( 'NONE',  ( -769.9999999999992042, 205.0000000000000568, -319.9999999999999432 ) ) ;
#41145=FACE_OUTER_BOUND ( 'NONE', #9136, .T. ) ;
#41163=DIRECTION ( 'NONE',  ( -1.000000000000000000, -0.000000000000000000, -0.000000000000000000 ) ) ;
#41174=VECTOR ( 'NONE', #32344, 1000.000000000000000 ) ;
#41196=LINE ( 'NONE', #9770, #11644 ) ;
#41241=AXIS2_PLACEMENT_3D ( 'NONE', #15509, #42988, #945 ) ;
#41275=FACE_OUTER_BOUND ( 'NONE', #3682, .T. ) ;
#41280=LINE ( 'NONE', #37809, #6069 ) ;
#41324=VERTEX_POINT ( 'NONE', #25361 ) ;
#41405=CARTESIAN_POINT ( 'NONE',  ( 265.7583438952258916, -600.0000000000000000, -320.0000000000000000 ) ) ;
#41411=DIRECTION ( 'NONE',  ( 1.000000000000000000, 0.000000000000000000, -0.000000000000000000 ) ) ;
#41440=ORIENTED_EDGE ( 'NONE', *, *, #2909, .T. ) ;
#41461=DIRECTION ( 'NONE',  ( 1.000000000000000000, -0.000000000000000000, -0.000000000000000000 ) ) ;
#41465=FACE_BOUND ( 'NONE', #25048, .T. ) ;
#41499=FACE_OUTER_BOUND ( 'NONE', #21094, .T. ) ;
#41557=VECTOR ( 'NONE', #23302, 1000.000000000000000 ) ;
#41572=LINE ( 'NONE', #17312, #20586 ) ;
#41610=EDGE_CURVE ( 'NONE', #637, #16382, #9039, .T. ) ;
#41617=( GEOMETRIC_REPRESENTATION_CONTEXT ( 3 ) GLOBAL_UNCERTAINTY_ASSIGNED_CONTEXT ( ( #30104 ) ) GLOBAL_UNIT_ASSIGNED_CONTEXT ( ( #24309, #2850, #6312 ) ) REPRESENTATION_CONTEXT ( 'NONE', 'WORKASPACE' ) );
#41641=CIRCLE ( 'NONE', #18767, 10.00000000000000888 ) ;
#41660=EDGE_LOOP ( 'NONE', ( #41440, #32408, #20527, #4234 ) ) ;
#41674=AXIS2_PLACEMENT_3D ( 'NONE', #33230, #12210, #5947 ) ;
#41680=DIRECTION ( 'NONE',  ( 5.551115123125783688E-16, -1.000000000000000000, 0.000000000000000000 ) ) ;
#41685=CARTESIAN_POINT ( 'NONE',  ( -769.9999999999992042, 205.0000000000000568, -360.0000000000000000 ) ) ;
#41700=VECTOR ( 'NONE', #44816, 1000.000000000000000 ) ;
#41712=ORIENTED_EDGE ( 'NONE', *, *, #45233, .T. ) ;
#41750=DIRECTION ( 'NONE',  ( -1.000000000000000000, 0.000000000000000000, 0.000000000000000000 ) ) ;
#41752=CARTESIAN_POINT ( 'NONE',  ( 180.7583438952259201, 394.6698570112193920, -244.9999999999999716 ) ) ;
#41770=VECTOR ( 'NONE', #1228, 1000.000000000000000 ) ;
#41817=AXIS2_PLACEMENT_3D ( 'NONE', #17712, #17015, #42179 ) ;
#41864=ADVANCED_FACE ( 'NONE', ( #1108 ), #1553, .F. ) ;
#41895=CYLINDRICAL_SURFACE ( 'NONE', #29945, 19.99999999999998934 ) ;
#41896=CARTESIAN_POINT ( 'NONE',  ( -769.9999999999992042, 205.0000000000000568, -360.0000000000000000 ) ) ;
#41914=CARTESIAN_POINT ( 'NONE',  ( -769.9999999999992042, 240.0000000000000853, -360.0000000000000000 ) ) ;
#41930=DIRECTION ( 'NONE',  ( 0.000000000000000000, 0.000000000000000000, 1.000000000000000000 ) ) ;
#41940=EDGE_CURVE ( 'NONE', #120, #34305, #26273, .T. ) ;
#41975=EDGE_CURVE ( 'NONE', #35390, #33022, #41280, .T. ) ;
#41982=DIRECTION ( 'NONE',  ( 0.000000000000000000, 0.000000000000000000, -1.000000000000000000 ) ) ;
#42000=ORIENTED_EDGE ( 'NONE', *, *, #11651, .T. ) ;
#42014=CARTESIAN_POINT ( 'NONE',  ( 879.9999999999992042, 430.0000000000002842, -244.9999999999999716 ) ) ;
#42059=ORIENTED_EDGE ( 'NONE', *, *, #11972, .T. ) ;
#42090=CARTESIAN_POINT ( 'NONE',  ( 829.9999999999992042, 579.9999999999998863, -360.0000000000000000 ) ) ;
#42113=CARTESIAN_POINT ( 'NONE',  ( 789.9999999999992042, 205.0000000000000568, -339.9999999999999432 ) ) ;
#42118=PLANE ( 'NONE',  #3270 ) ;
#42153=CARTESIAN_POINT ( 'NONE',  ( 1238.921997096861332, 430.0000000000002842, -244.9999999999999716 ) ) ;
#42162=STYLED_ITEM('',(#45744),#17465);
#42179=DIRECTION ( 'NONE',  ( 1.000000000000000000, 0.000000000000000000, 0.000000000000000000 ) ) ;
#42213=EDGE_CURVE ( 'NONE', #18941, #7747, #30190, .T. ) ;
#42218=LINE ( 'NONE', #34605, #35733 ) ;
#42223=EDGE_CURVE ( 'NONE', #6383, #10220, #5711, .T. ) ;
#42263=VERTEX_POINT ( 'NONE', #33882 ) ;
#42276=VECTOR ( 'NONE', #35514, 1000.000000000000000 ) ;
#42335=DIRECTION ( 'NONE',  ( 0.000000000000000000, 0.000000000000000000, -1.000000000000000000 ) ) ;
#42413=DIRECTION ( 'NONE',  ( 1.000000000000000000, -0.000000000000000000, -0.000000000000000000 ) ) ;
#42432=VECTOR ( 'NONE', #3805, 1000.000000000000000 ) ;
#42460=CARTESIAN_POINT ( 'NONE',  ( 1238.921997096861332, 430.0000000000002842, -320.0000000000000568 ) ) ;
#42466=CARTESIAN_POINT ( 'NONE',  ( 115.7583438952258774, -600.0000000000000000, -244.9999999999999716 ) ) ;
#42502=PRODUCT_DEFINITION_SHAPE ( 'NONE', 'NONE',  #28146 ) ;
#42510=EDGE_CURVE ( 'NONE', #17206, #12447, #28224, .T. ) ;
#42547=EDGE_CURVE ( 'NONE', #45022, #6383, #20923, .T. ) ;
#42569=ORIENTED_EDGE ( 'NONE', *, *, #38186, .T. ) ;
#42638=CYLINDRICAL_SURFACE ( 'NONE', #435, 10.00000000000000888 ) ;
#42646=LINE ( 'NONE', #42861, #16756 ) ;
#42680=ORIENTED_EDGE ( 'NONE', *, *, #38536, .F. ) ;
#42690=CIRCLE ( 'NONE', #25711, 20.00000000000001776 ) ;
#42739=CARTESIAN_POINT ( 'NONE',  ( 190.7583438952259485, 290.0000000000001137, -274.9999999999999432 ) ) ;
#42743=ADVANCED_FACE ( 'NONE', ( #34789 ), #35252, .F. ) ;
#42759=PLANE ( 'NONE',  #29102 ) ;
#42809=EDGE_LOOP ( 'NONE', ( #5723, #8428, #9154, #30110 ) ) ;
#42812=DIRECTION ( 'NONE',  ( 0.000000000000000000, 0.000000000000000000, -1.000000000000000000 ) ) ;
#42820=DIRECTION ( 'NONE',  ( -1.000000000000000000, 0.000000000000000000, 0.000000000000000000 ) ) ;
#42861=CARTESIAN_POINT ( 'NONE',  ( -180.7583438952258348, 394.6698570112193920, -274.9999999999999432 ) ) ;
#42862=CARTESIAN_POINT ( 'NONE',  ( -181.9156952255813735, 290.0000000000001137, -274.9999999999999432 ) ) ;
#42866=FACE_OUTER_BOUND ( 'NONE', #40622, .T. ) ;
#42899=VERTEX_POINT ( 'NONE', #19074 ) ;
#42960=ORIENTED_EDGE ( 'NONE', *, *, #34333, .F. ) ;
#42985=DIRECTION ( 'NONE',  ( 1.000000000000000000, -0.000000000000000000, -0.000000000000000000 ) ) ;
#42988=DIRECTION ( 'NONE',  ( 0.000000000000000000, 0.000000000000000000, 1.000000000000000000 ) ) ;
#43007=AXIS2_PLACEMENT_3D ( 'NONE', #10535, #7544, #31780 ) ;
#43009=ORIENTED_EDGE ( 'NONE', *, *, #17569, .T. ) ;
#43032=CARTESIAN_POINT ( 'NONE',  ( 355.8971257818259915, 290.0000000000001137, -244.9999999999999716 ) ) ;
#43052=CARTESIAN_POINT ( 'NONE',  ( -879.9999999999992042, 240.0000000000000568, -244.9999999999999716 ) ) ;
#43076=ORIENTED_EDGE ( 'NONE', *, *, #43599, .T. ) ;
#43078=EDGE_CURVE ( 'NONE', #42263, #5389, #2644, .T. ) ;
#43082=DIRECTION ( 'NONE',  ( -0.000000000000000000, -0.000000000000000000, 1.000000000000000000 ) ) ;
#43216=CYLINDRICAL_SURFACE ( 'NONE', #18056, 10.00000000000000888 ) ;
#43222=AXIS2_PLACEMENT_3D ( 'NONE', #29235, #7530, #35238 ) ;
#43247=ORIENTED_EDGE ( 'NONE', *, *, #44758, .T. ) ;
#43282=VECTOR ( 'NONE', #28139, 1000.000000000000000 ) ;
#43347=EDGE_CURVE ( 'NONE', #21916, #38320, #9799, .T. ) ;
#43379=DIRECTION ( 'NONE',  ( -0.000000000000000000, -1.000000000000000000, -0.000000000000000000 ) ) ;
#43383=DIRECTION ( 'NONE',  ( 5.551115123125783688E-16, -1.000000000000000000, 0.000000000000000000 ) ) ;
#43403=ORIENTED_EDGE ( 'NONE', *, *, #11150, .F. ) ;
#43413=ORIENTED_EDGE ( 'NONE', *, *, #11931, .T. ) ;
#43416=AXIS2_PLACEMENT_3D ( 'NONE', #15399, #29480, #43552 ) ;
#43485=CARTESIAN_POINT ( 'NONE',  ( -769.9999999999992042, 205.0000000000000568, -319.9999999999999432 ) ) ;
#43537=DIRECTION ( 'NONE',  ( -1.000000000000000000, 0.000000000000000000, -0.000000000000000000 ) ) ;
#43552=DIRECTION ( 'NONE',  ( 0.000000000000000000, 0.000000000000000000, 1.000000000000000000 ) ) ;
#43589=LINE ( 'NONE', #26024, #29203 ) ;
#43591=LINE ( 'NONE', #3894, #1966 ) ;
#43599=EDGE_CURVE ( 'NONE', #120, #3087, #36277, .T. ) ;
#43600=ORIENTED_EDGE ( 'NONE', *, *, #33454, .T. ) ;
#43632=ORIENTED_EDGE ( 'NONE', *, *, #10271, .F. ) ;
#43685=VERTEX_POINT ( 'NONE', #193 ) ;
#43711=DIRECTION ( 'NONE',  ( 0.000000000000000000, -0.000000000000000000, -1.000000000000000000 ) ) ;
#43746=CARTESIAN_POINT ( 'NONE',  ( 769.9999999999992042, 205.0000000000000568, -360.0000000000000000 ) ) ;
#43761=LINE ( 'NONE', #37297, #12083 ) ;
#43790=ORIENTED_EDGE ( 'NONE', *, *, #4385, .T. ) ;
#43805=LINE ( 'NONE', #9166, #26301 ) ;
#43832=DIRECTION ( 'NONE',  ( -1.000000000000000000, -0.000000000000000000, 0.000000000000000000 ) ) ;
#43836=EDGE_CURVE ( 'NONE', #7747, #12562, #39011, .T. ) ;
#43865=EDGE_CURVE ( 'NONE', #29001, #1656, #28829, .T. ) ;
#43907=ORIENTED_EDGE ( 'NONE', *, *, #9431, .F. ) ;
#43915=ORIENTED_EDGE ( 'NONE', *, *, #40244, .F. ) ;
#43918=VECTOR ( 'NONE', #28832, 1000.000000000000000 ) ;
#43923=ADVANCED_FACE ( 'NONE', ( #44514 ), #8742, .F. ) ;
#43929=DIRECTION ( 'NONE',  ( -0.000000000000000000, 1.000000000000000000, -0.000000000000000000 ) ) ;
#43933=LINE ( 'NONE', #36997, #19465 ) ;
#43952=AXIS2_PLACEMENT_3D ( 'NONE', #44904, #19958, #3081 ) ;
#43989=DIRECTION ( 'NONE',  ( 0.000000000000000000, 0.000000000000000000, -1.000000000000000000 ) ) ;
#43996=VECTOR ( 'NONE', #27291, 1000.000000000000000 ) ;
#44013=DIRECTION ( 'NONE',  ( -1.000000000000000000, -0.000000000000000000, -0.000000000000000000 ) ) ;
#44058=VECTOR ( 'NONE', #28559, 1000.000000000000000 ) ;
#44081=EDGE_CURVE ( 'NONE', #10220, #45456, #13114, .T. ) ;
#44099=LINE ( 'NONE', #12463, #24839 ) ;
#44110=LINE ( 'NONE', #12474, #19567 ) ;
#44144=VERTEX_POINT ( 'NONE', #23480 ) ;
#44202=ORIENTED_EDGE ( 'NONE', *, *, #26039, .T. ) ;
#44233=AXIS2_PLACEMENT_3D ( 'NONE', #19729, #36207, #14974 ) ;
#44245=LINE ( 'NONE', #19523, #25480 ) ;
#44276=LINE ( 'NONE', #12414, #44773 ) ;
#44279=CARTESIAN_POINT ( 'NONE',  ( -180.7583438952258348, 394.6698570112193920, -274.9999999999999432 ) ) ;
#44345=DIRECTION ( 'NONE',  ( -1.000000000000000000, 0.000000000000000000, 0.000000000000000000 ) ) ;
#44362=CARTESIAN_POINT ( 'NONE',  ( -115.7583438952258774, 290.0000000000001137, -320.0000000000000568 ) ) ;
#44381=CARTESIAN_POINT ( 'NONE',  ( 789.9999999999992042, 240.0000000000000568, -319.9999999999999432 ) ) ;
#44416=EDGE_CURVE ( 'NONE', #21150, #17206, #31101, .T. ) ;
#44440=LINE ( 'NONE', #12129, #23387 ) ;
#44450=EDGE_CURVE ( 'NONE', #13136, #23168, #22413, .T. ) ;
#44514=FACE_OUTER_BOUND ( 'NONE', #10932, .T. ) ;
#44524=VECTOR ( 'NONE', #29571, 1000.000000000000000 ) ;
#44530=ORIENTED_EDGE ( 'NONE', *, *, #11726, .F. ) ;
#44537=VECTOR ( 'NONE', #14656, 1000.000000000000000 ) ;
#44582=DIRECTION ( 'NONE',  ( 0.000000000000000000, 1.000000000000000000, 3.700743415417198493E-16 ) ) ;
#44593=EDGE_LOOP ( 'NONE', ( #29425, #21551, #44788, #24995, #7261, #14204, #35970, #5223, #28479, #21696, #9451, #10756, #30927, #16765, #13414, #43907, #42000, #43600 ) ) ;
#44604=ORIENTED_EDGE ( 'NONE', *, *, #29307, .T. ) ;
#44609=VERTEX_POINT ( 'NONE', #4085 ) ;
#44613=VERTEX_POINT ( 'NONE', #8226 ) ;
#44645=LINE ( 'NONE', #42090, #2594 ) ;
#44654=DIRECTION ( 'NONE',  ( 0.000000000000000000, 0.000000000000000000, 1.000000000000000000 ) ) ;
#44657=AXIS2_PLACEMENT_3D ( 'NONE', #31086, #45183, #10082 ) ;
#44745=DIRECTION ( 'NONE',  ( -1.000000000000000000, -0.000000000000000000, -0.000000000000000000 ) ) ;
#44758=EDGE_CURVE ( 'NONE', #36817, #6928, #4532, .T. ) ;
#44773=VECTOR ( 'NONE', #12633, 1000.000000000000000 ) ;
#44788=ORIENTED_EDGE ( 'NONE', *, *, #43347, .T. ) ;
#44800=LINE ( 'NONE', #33928, #19660 ) ;
#44804=ORIENTED_EDGE ( 'NONE', *, *, #41610, .F. ) ;
#44816=DIRECTION ( 'NONE',  ( -0.000000000000000000, -6.938893903907222461E-16, 1.000000000000000000 ) ) ;
#44836=DIRECTION ( 'NONE',  ( -0.000000000000000000, 1.000000000000000000, -0.000000000000000000 ) ) ;
#44856=ORIENTED_EDGE ( 'NONE', *, *, #28934, .F. ) ;
#44903=CARTESIAN_POINT ( 'NONE',  ( 181.9156952255813735, 290.0000000000001137, -274.9999999999999432 ) ) ;
#44904=CARTESIAN_POINT ( 'NONE',  ( 794.9999999999993179, 205.0000000000000568, -255.0000000000000000 ) ) ;
#44934=EDGE_CURVE ( 'NONE', #45022, #42263, #616, .T. ) ;
#44949=ORIENTED_EDGE ( 'NONE', *, *, #7247, .F. ) ;
#44969=AXIS2_PLACEMENT_3D ( 'NONE', #24089, #35185, #27121 ) ;
#44978=ORIENTED_EDGE ( 'NONE', *, *, #15141, .T. ) ;
#44986=DIRECTION ( 'NONE',  ( -1.000000000000000000, -0.000000000000000000, -0.000000000000000000 ) ) ;
#45022=VERTEX_POINT ( 'NONE', #25982 ) ;
#45035=EDGE_CURVE ( 'NONE', #39971, #45077, #43761, .T. ) ;
#45060=UNCERTAINTY_MEASURE_WITH_UNIT (LENGTH_MEASURE( 1.000000000000000082E-05 ), #37692, 'distance_accuracy_value', 'NONE');
#45077=VERTEX_POINT ( 'NONE', #4986 ) ;
#45093=CYLINDRICAL_SURFACE ( 'NONE', #16574, 10.00000000000000888 ) ;
#45095=CARTESIAN_POINT ( 'NONE',  ( 794.9999999999993179, 205.0000000000000568, -265.0000000000000000 ) ) ;
#45107=CARTESIAN_POINT ( 'NONE',  ( 769.9999999999992042, 205.0000000000000568, -350.0000000000000000 ) ) ;
#45115=VERTEX_POINT ( 'NONE', #15601 ) ;
#45117=DIRECTION ( 'NONE',  ( 8.326672684688676025E-16, -1.000000000000000000, 0.000000000000000000 ) ) ;
#45125=ORIENTED_EDGE ( 'NONE', *, *, #25197, .T. ) ;
#45163=ORIENTED_EDGE ( 'NONE', *, *, #1735, .T. ) ;
#45183=DIRECTION ( 'NONE',  ( 1.000000000000000000, 0.000000000000000000, -0.000000000000000000 ) ) ;
#45206=ORIENTED_EDGE ( 'NONE', *, *, #114, .T. ) ;
#45233=EDGE_CURVE ( 'NONE', #22309, #34504, #2191, .T. ) ;
#45250=VECTOR ( 'NONE', #29735, 1000.000000000000000 ) ;
#45301=ADVANCED_FACE ( 'NONE', ( #8900 ), #22967, .F. ) ;
#45303=ORIENTED_EDGE ( 'NONE', *, *, #13183, .F. ) ;
#45314=VECTOR ( 'NONE', #28204, 1000.000000000000000 ) ;
#45323=LINE ( 'NONE', #38867, #380 ) ;
#45341=CARTESIAN_POINT ( 'NONE',  ( -769.9999999999992042, 205.0000000000000568, -350.0000000000000000 ) ) ;
#45347=EDGE_LOOP ( 'NONE', ( #2669, #8657, #4849, #19375 ) ) ;
#45361=FACE_OUTER_BOUND ( 'NONE', #28643, .T. ) ;
#45363=ORIENTED_EDGE ( 'NONE', *, *, #25547, .T. ) ;
#45394=CARTESIAN_POINT ( 'NONE',  ( 181.9156952255813735, 290.0000000000001137, -274.9999999999999432 ) ) ;
#45403=DIRECTION ( 'NONE',  ( -1.000000000000000000, -0.000000000000000000, -0.000000000000000000 ) ) ;
#45412=CIRCLE ( 'NONE', #4815, 20.00000000000001776 ) ;
#45424=ORIENTED_EDGE ( 'NONE', *, *, #19317, .F. ) ;
#45456=VERTEX_POINT ( 'NONE', #17191 ) ;
#45461=ORIENTED_EDGE ( 'NONE', *, *, #20695, .F. ) ;
#45491=VERTEX_POINT ( 'NONE', #37760 ) ;
#45522=EDGE_CURVE ( 'NONE', #18651, #36310, #6109, .T. ) ;
#45525=LINE ( 'NONE', #20566, #10204 ) ;
#45556=FACE_OUTER_BOUND ( 'NONE', #16712, .T. ) ;
#45586=ORIENTED_EDGE ( 'NONE', *, *, #41610, .T. ) ;
#45608=DIRECTION ( 'NONE',  ( 0.000000000000000000, 0.000000000000000000, 1.000000000000000000 ) ) ;
#45631=LINE ( 'NONE', #6804, #40941 ) ;
#45655=DIRECTION ( 'NONE',  ( 0.000000000000000000, 1.000000000000000000, 0.000000000000000000 ) ) ;
#45701=VECTOR ( 'NONE', #25882, 1000.000000000000000 ) ;
#45738=COLOUR_RGB('Dark Blue',0.08,0.2,0.34);
#45739=FILL_AREA_STYLE_COLOUR('',#45738);
#45740=FILL_AREA_STYLE('',(#45739));
#45741=SURFACE_STYLE_FILL_AREA(#45740);
#45742=SURFACE_SIDE_STYLE('',(#45741));
#45743=SURFACE_STYLE_USAGE(.BOTH.,#45742);
#45744=PRESENTATION_STYLE_ASSIGNMENT((#45743));
ENDSEC;
END-ISO-10303-21;
